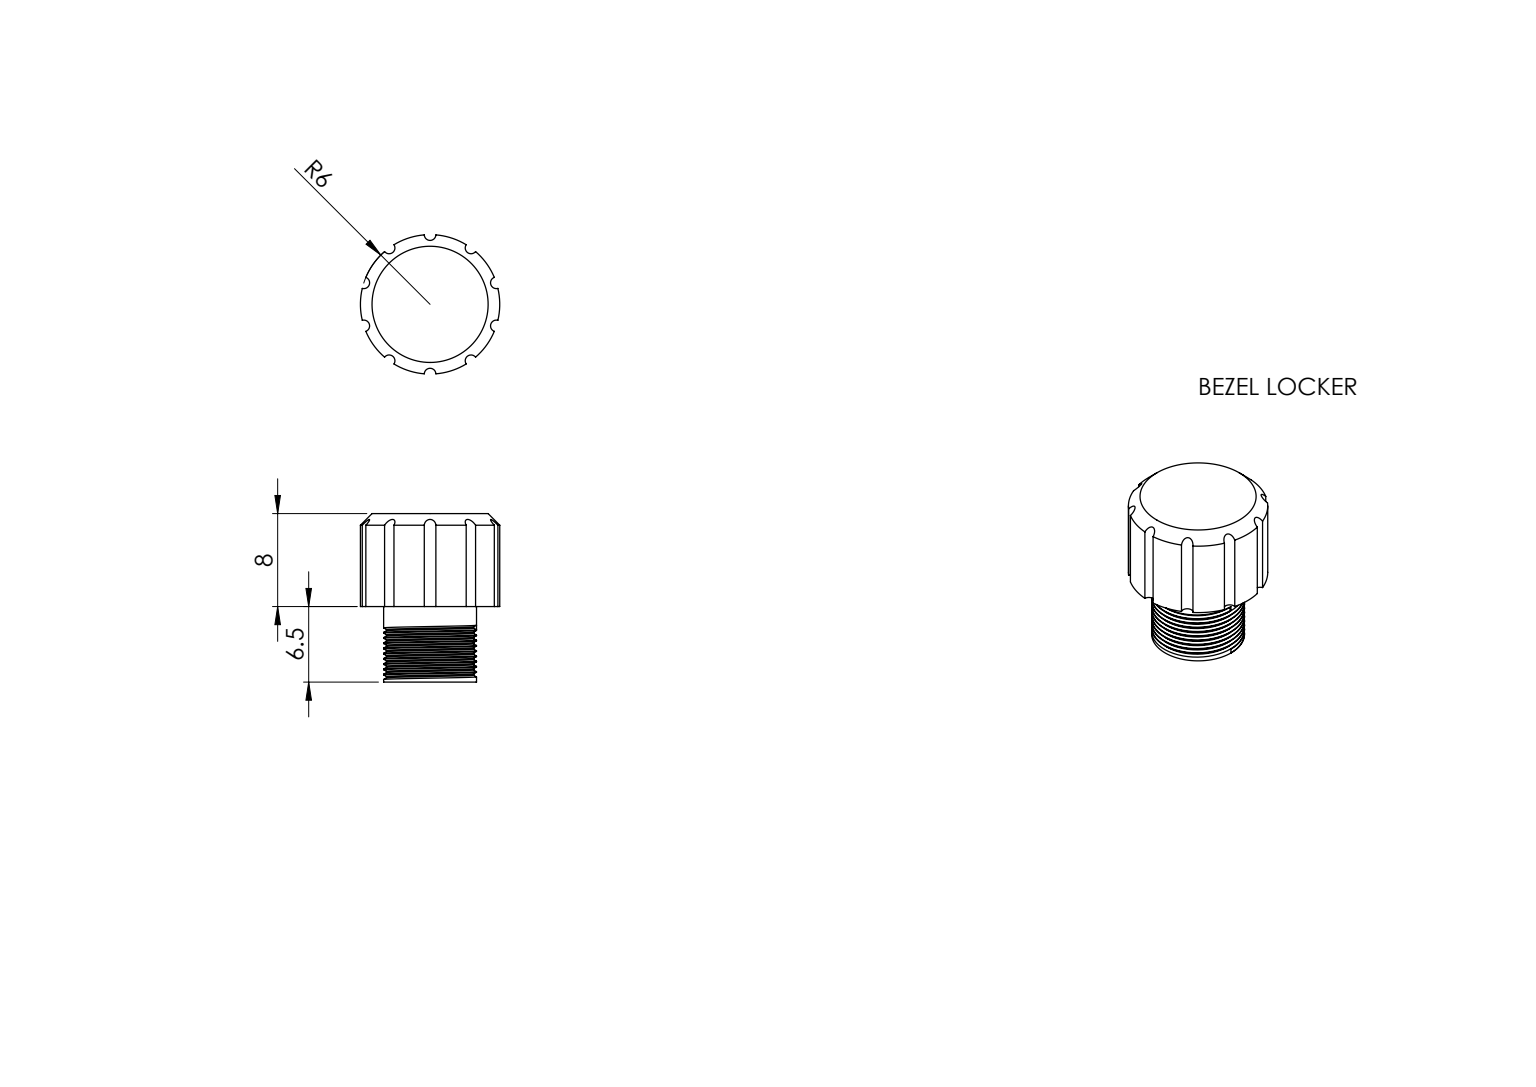
ISO-10303-21;
HEADER;
FILE_DESCRIPTION (('STEP AP214'),
    '1' );
FILE_NAME ('bezel locker.step',
    '2026-10-26T12:50:16',
    ( '' ),
    ( '' ),
    'SwSTEP 2.0',
    'SolidWorks 2026',
    '' );
FILE_SCHEMA (( 'AUTOMOTIVE_DESIGN' ));
ENDSEC;

DATA;
#10=DIRECTION ( 'NONE',  ( 0.000000000000000000, 0.000000000000000000, -1.000000000000000000 ) ) ;
#19=CARTESIAN_POINT ( 'NONE',  ( 3.469446951953614189E-15, 35.50000000000000711, 8.999999999999992895 ) ) ;
#32=VERTEX_POINT ( 'NONE', #17367 ) ;
#40=CARTESIAN_POINT ( 'NONE',  ( 7.901901826148023498E-15, 27.53124999877097068, 12.99999999999999112 ) ) ;
#46=CONICAL_SURFACE ( 'NONE', #10212, 5.000000000000000888, 0.7853981633974445042 ) ;
#53=CARTESIAN_POINT ( 'NONE',  ( -3.999999999999996447, 29.63124999877097210, 6.690598923241487306 ) ) ;
#61=ADVANCED_FACE ( 'NONE', ( #4267 ), #12239, .F. ) ;
#62=ORIENTED_EDGE ( 'NONE', *, *, #6026, .F. ) ;
#69=CARTESIAN_POINT ( 'NONE',  ( -3.756430356249997882, 29.45312499938549067, 11.16877607737301048 ) ) ;
#73=CARTESIAN_POINT ( 'NONE',  ( 4.000000000000002665, 27.21250000000000568, 11.30940107675849760 ) ) ;
#87=CARTESIAN_POINT ( 'NONE',  ( 3.756430356250004987, 25.19687499938549280, 8.999999999999992895 ) ) ;
#92=CARTESIAN_POINT ( 'NONE',  ( 4.006172263299091013E-15, 27.16562499938547859, 4.662447845253954171 ) ) ;
#93=ORIENTED_EDGE ( 'NONE', *, *, #14257, .T. ) ;
#101=CARTESIAN_POINT ( 'NONE',  ( 3.756430356250002323, 27.35312499938548569, 11.16877607737301226 ) ) ;
#113=EDGE_CURVE ( 'NONE', #22373, #14800, #20983, .T. ) ;
#114=DIRECTION ( 'NONE',  ( -0.000000000000000000, -1.000000000000000000, -0.000000000000000000 ) ) ;
#115=CARTESIAN_POINT ( 'NONE',  ( 3.718542035834364277E-15, 25.11250000000000782, 4.999999999999992006 ) ) ;
#118=CARTESIAN_POINT ( 'NONE',  ( -5.395002858709908367, 38.91217497027906802, 10.45656796931105426 ) ) ;
#121=AXIS2_PLACEMENT_3D ( 'NONE', #5758, #23946, #12025 ) ;
#123=CARTESIAN_POINT ( 'NONE',  ( 3.469446951953614189E-15, 35.50000000000000711, 4.999999999999992006 ) ) ;
#124=CARTESIAN_POINT ( 'NONE',  ( 3.370160183775990248, 38.97860908142764913, 13.37397733810513856 ) ) ;
#126=CARTESIAN_POINT ( 'NONE',  ( 2.000000000000005329, 26.81874999877097210, 5.535898384862238508 ) ) ;
#127=CARTESIAN_POINT ( 'NONE',  ( 3.469446951953614189E-15, 35.50000000000000711, 4.999999999999992006 ) ) ;
#139=CARTESIAN_POINT ( 'NONE',  ( -1.878215178124998275, 25.89062499938549067, 12.25316411605951927 ) ) ;
#144=EDGE_CURVE ( 'NONE', #7410, #22395, #341, .T. ) ;
#155=CARTESIAN_POINT ( 'NONE',  ( 1.071796769724497222, 28.00134618820329990, 12.99999999999998757 ) ) ;
#166=ORIENTED_EDGE ( 'NONE', *, *, #16755, .F. ) ;
#185=CARTESIAN_POINT ( 'NONE',  ( -1.878215178124994722, 25.40312499938548996, 5.746835883940462963 ) ) ;
#189=CARTESIAN_POINT ( 'NONE',  ( -3.999999999999996447, 29.23750000000001137, 6.690598923241487306 ) ) ;
#194=LINE ( 'NONE', #20580, #24770 ) ;
#196=FACE_OUTER_BOUND ( 'NONE', #24755, .T. ) ;
#200=CARTESIAN_POINT ( 'NONE',  ( -1.859271017917182139E-15, 26.46249999999999858, 4.999999999999991118 ) ) ;
#204=EDGE_CURVE ( 'NONE', #4422, #2251, #3256, .T. ) ;
#216=CARTESIAN_POINT ( 'NONE',  ( -1.878215178124999829, 26.90312499938548640, 12.25316411605951927 ) ) ;
#224=CARTESIAN_POINT ( 'NONE',  ( -3.756430356249998326, 28.10312499938548569, 11.16877607737301226 ) ) ;
#228=CARTESIAN_POINT ( 'NONE',  ( -3.999999999999999112, 28.35624999877097707, 11.30940107675849404 ) ) ;
#236=CARTESIAN_POINT ( 'NONE',  ( -3.999999999999996447, 26.51874999877097494, 8.999999999999992895 ) ) ;
#241=DIRECTION ( 'NONE',  ( -0.000000000000000000, -1.000000000000000000, -0.000000000000000000 ) ) ;
#247=CARTESIAN_POINT ( 'NONE',  ( -4.000000000000001776, 29.21874999877097068, 8.999999999999992895 ) ) ;
#251=CARTESIAN_POINT ( 'NONE',  ( 4.000000000000002665, 26.70624999877097849, 11.30940107675849760 ) ) ;
#264=CARTESIAN_POINT ( 'NONE',  ( 1.878215178125001605, 27.76562499938548711, 12.25316411605952283 ) ) ;
#302=DIRECTION ( 'NONE',  ( 0.000000000000000000, 0.000000000000000000, -1.000000000000000000 ) ) ;
#305=ORIENTED_EDGE ( 'NONE', *, *, #21565, .F. ) ;
#307=CARTESIAN_POINT ( 'NONE',  ( -3.756430356250002323, 27.31562499938548783, 11.16877607737301226 ) ) ;
#322=CARTESIAN_POINT ( 'NONE',  ( -3.999999999999996447, 28.86250000000000071, 11.30940107675849404 ) ) ;
#333=ORIENTED_EDGE ( 'NONE', *, *, #23959, .T. ) ;
#336=CARTESIAN_POINT ( 'NONE',  ( -1.878215178124998275, 28.25312499938548783, 12.25316411605951927 ) ) ;
#340=EDGE_CURVE ( 'NONE', #19215, #8133, #14856, .T. ) ;
#341=LINE ( 'NONE', #20331, #16761 ) ;
#345=VERTEX_POINT ( 'NONE', #10775 ) ;
#348=CARTESIAN_POINT ( 'NONE',  ( -1.878215178124999829, 29.04062499938549280, 12.25316411605951927 ) ) ;
#352=CIRCLE ( 'NONE', #6610, 6.000000000000000000 ) ;
#355=AXIS2_PLACEMENT_3D ( 'NONE', #19379, #17425, #11406 ) ;
#384=ADVANCED_FACE ( 'NONE', ( #5558 ), #46, .T. ) ;
#386=CARTESIAN_POINT ( 'NONE',  ( -1.878215178124998275, 25.55312499938549564, 12.25316411605951927 ) ) ;
#388=AXIS2_PLACEMENT_3D ( 'NONE', #11786, #19763, #1858 ) ;
#389=EDGE_CURVE ( 'NONE', #6543, #18698, #23590, .T. ) ;
#398=CARTESIAN_POINT ( 'NONE',  ( 3.918623196469464443, 31.50000000000000000, 4.456389954662531849 ) ) ;
#409=CARTESIAN_POINT ( 'NONE',  ( 2.000000000000003553, 27.71874999877097778, 5.535898384862238508 ) ) ;
#415=EDGE_LOOP ( 'NONE', ( #19879, #25527, #12734, #3697 ) ) ;
#418=FACE_OUTER_BOUND ( 'NONE', #25244, .T. ) ;
#445=CARTESIAN_POINT ( 'NONE',  ( -1.878215178124994722, 26.75312499938549138, 5.746835883940462963 ) ) ;
#458=CARTESIAN_POINT ( 'NONE',  ( 3.469446951953614189E-15, 39.50000000000000000, 8.999999999999992895 ) ) ;
#462=LINE ( 'NONE', #12609, #10063 ) ;
#463=DIRECTION ( 'NONE',  ( -0.000000000000000000, -1.000000000000000000, -0.000000000000000000 ) ) ;
#475=CARTESIAN_POINT ( 'NONE',  ( 5.255164635687713748, 38.99989214654019065, 10.62496012790605704 ) ) ;
#479=CARTESIAN_POINT ( 'NONE',  ( -1.878215178124998275, 28.10312499938548925, 5.746835883940462963 ) ) ;
#482=CARTESIAN_POINT ( 'NONE',  ( 3.469446951953614189E-15, 39.50000000000000000, 8.999999999999992895 ) ) ;
#486=VERTEX_POINT ( 'NONE', #5677 ) ;
#488=CARTESIAN_POINT ( 'NONE',  ( 1.878215178125003382, 28.36562499938548498, 5.746835883940462963 ) ) ;
#518=AXIS2_PLACEMENT_3D ( 'NONE', #19501, #15217, #9328 ) ;
#524=CARTESIAN_POINT ( 'NONE',  ( 1.487416814333745711E-14, 28.03750000000001208, 12.99999999999999289 ) ) ;
#525=CARTESIAN_POINT ( 'NONE',  ( 1.878215178125005158, 25.77812499938548996, 5.746835883940462963 ) ) ;
#530=CARTESIAN_POINT ( 'NONE',  ( -3.481870629348635671, 38.92501902593045315, 4.645898033751316270 ) ) ;
#556=AXIS2_PLACEMENT_3D ( 'NONE', #19, #15717, #3807 ) ;
#558=DIRECTION ( 'NONE',  ( 0.000000000000000000, 1.000000000000000000, 0.000000000000000000 ) ) ;
#578=CARTESIAN_POINT ( 'NONE',  ( -1.878215178124999829, 26.90312499938548640, 12.25316411605951927 ) ) ;
#587=STYLED_ITEM('',(#25907),#5394);
#600=CARTESIAN_POINT ( 'NONE',  ( -0.4995657836784015426, 38.49999999999999289, 3.020833333333323267 ) ) ;
#601=CARTESIAN_POINT ( 'NONE',  ( 4.000000000000002665, 25.80624999877096926, 11.30940107675849760 ) ) ;
#604=EDGE_CURVE ( 'NONE', #23841, #1729, #1999, .T. ) ;
#605=CARTESIAN_POINT ( 'NONE',  ( 5.563387625853419394, 38.77026726007181878, 10.37110993082982979 ) ) ;
#609=CARTESIAN_POINT ( 'NONE',  ( 3.756430356250002323, 27.46562499938548640, 11.16877607737301403 ) ) ;
#614=CARTESIAN_POINT ( 'NONE',  ( 3.526711513754818395, 29.50000000000000000, 4.145898033750289535 ) ) ;
#618=CARTESIAN_POINT ( 'NONE',  ( 3.756430356250004987, 27.84062499938548640, 8.999999999999992895 ) ) ;
#631=FACE_OUTER_BOUND ( 'NONE', #5269, .T. ) ;
#633=CARTESIAN_POINT ( 'NONE',  ( -3.999999999999998224, 25.61874999877097281, 8.999999999999992895 ) ) ;
#639=DIRECTION ( 'NONE',  ( 0.000000000000000000, 1.000000000000000000, -0.000000000000000000 ) ) ;
#656=DIRECTION ( 'NONE',  ( 0.000000000000000000, -1.000000000000000000, -0.000000000000000000 ) ) ;
#699=CARTESIAN_POINT ( 'NONE',  ( 3.756430356250004543, 28.81562499938548783, 11.16877607737301226 ) ) ;
#704=CARTESIAN_POINT ( 'NONE',  ( -1.071796769724485232, 27.77634618820331269, 4.999999999999992006 ) ) ;
#711=LINE ( 'NONE', #8815, #3315 ) ;
#718=CARTESIAN_POINT ( 'NONE',  ( 0.000000000000000000, 25.73124999877097352, 13.61880215351699874 ) ) ;
#719=CARTESIAN_POINT ( 'NONE',  ( 3.959305671612554781E-15, 35.50000000000000711, 12.99999999999999289 ) ) ;
#735=CARTESIAN_POINT ( 'NONE',  ( 3.756430356250003211, 26.04062499938548925, 8.999999999999992895 ) ) ;
#751=ORIENTED_EDGE ( 'NONE', *, *, #3136, .F. ) ;
#759=CARTESIAN_POINT ( 'NONE',  ( 4.000000000000001776, 29.89374999877097139, 8.999999999999992895 ) ) ;
#765=CARTESIAN_POINT ( 'NONE',  ( -3.756430356249996105, 25.44062499938548783, 6.831223922626973533 ) ) ;
#797=ORIENTED_EDGE ( 'NONE', *, *, #18776, .F. ) ;
#804=LINE ( 'NONE', #24741, #11411 ) ;
#810=DIRECTION ( 'NONE',  ( -0.000000000000000000, -1.000000000000000000, 0.000000000000000000 ) ) ;
#813=CARTESIAN_POINT ( 'NONE',  ( -3.999999999999996447, 29.63124999877097210, 6.690598923241487306 ) ) ;
#816=DIRECTION ( 'NONE',  ( 0.000000000000000000, 0.000000000000000000, 1.000000000000000000 ) ) ;
#819=CARTESIAN_POINT ( 'NONE',  ( 1.878215178125003382, 28.02812499938548996, 5.746835883940462963 ) ) ;
#847=CARTESIAN_POINT ( 'NONE',  ( -3.999999999999996447, 26.48124999877096997, 6.690598923241487306 ) ) ;
#849=CARTESIAN_POINT ( 'NONE',  ( 5.428131658003001903, 38.61087488181073724, 11.28411968614168615 ) ) ;
#855=VERTEX_POINT ( 'NONE', #17017 ) ;
#864=CARTESIAN_POINT ( 'NONE',  ( -3.756430356249996549, 26.67812499938548854, 6.831223922626973533 ) ) ;
#865=AXIS2_PLACEMENT_3D ( 'NONE', #18096, #5921, #4344 ) ;
#866=CARTESIAN_POINT ( 'NONE',  ( 1.071796769724492782, 26.44240381056766509, 4.999999999999989342 ) ) ;
#867=CARTESIAN_POINT ( 'NONE',  ( 3.756430356250002323, 28.25312499938548783, 11.16877607737301226 ) ) ;
#882=AXIS2_PLACEMENT_3D ( 'NONE', #14642, #16737, #24706 ) ;
#884=CARTESIAN_POINT ( 'NONE',  ( -3.999999999999996447, 25.65624999877097068, 11.30940107675849404 ) ) ;
#902=CARTESIAN_POINT ( 'NONE',  ( -3.756430356249994773, 28.17812499938548854, 8.999999999999992895 ) ) ;
#924=CARTESIAN_POINT ( 'NONE',  ( 4.648177544792955347E-16, 26.68750000000000711, 12.99999999999999289 ) ) ;
#930=VERTEX_POINT ( 'NONE', #7833 ) ;
#948=AXIS2_PLACEMENT_3D ( 'NONE', #2206, #241, #4289 ) ;
#958=AXIS2_PLACEMENT_3D ( 'NONE', #19324, #9263, #17252 ) ;
#960=ORIENTED_EDGE ( 'NONE', *, *, #11857, .T. ) ;
#981=ORIENTED_EDGE ( 'NONE', *, *, #3136, .T. ) ;
#982=CARTESIAN_POINT ( 'NONE',  ( 2.000000000000000000, 25.76874999877097139, 12.46410161513774817 ) ) ;
#996=LINE ( 'NONE', #14734, #15134 ) ;
#1000=CARTESIAN_POINT ( 'NONE',  ( -1.878215178124999829, 29.04062499938549280, 12.25316411605951927 ) ) ;
#1020=DIRECTION ( 'NONE',  ( -0.000000000000000000, -1.000000000000000000, -0.000000000000000000 ) ) ;
#1031=CARTESIAN_POINT ( 'NONE',  ( 3.756430356250004543, 28.81562499938548783, 11.16877607737301226 ) ) ;
#1035=EDGE_CURVE ( 'NONE', #18677, #23884, #21970, .T. ) ;
#1036=CARTESIAN_POINT ( 'NONE',  ( -3.100818392631252696, 38.96327129008100343, 4.412772063012910806 ) ) ;
#1054=EDGE_LOOP ( 'NONE', ( #15352, #6511, #21097, #21569 ) ) ;
#1063=( BOUNDED_SURFACE ( )  B_SPLINE_SURFACE ( 1, 2, ( 
 ( #4499, #12474, #18900, #2547, #4375, #12621, #12354, #10517, #18514, #718, #982, #601, #16550, #14846, #24780, #24255, #24509, #6591, #24638, #16670, #10766, #20594, #2680, #6726, #14718, #4778, #20723, #4895, #18755, #847, #8827, #6863, #12871, #11156, #21500, #11290, #17201, #15234, #13531, #5029, #25173, #22943, #11037, #23082, #11550, #16938, #23320, #23458, #9347, #23198, #21375, #9466, #19016, #13398, #15350, #3188, #5168, #19137, #24908, #21231, #19517, #13009, #7121, #9211, #7253, #1100, #25294, #7497, #13259, #3314, #15490, #20993, #6984, #15107, #3454, #5283, #17329, #11428, #14966, #9076, #3070, #17059, #5547, #19402, #7373, #3579, #25030, #8963, #19270, #1372, #13146, #5411, #21110, #1493, #1229, #17443, #25410, #13779, #8026, #21886, #9590, #21616, #23589, #11817, #25552, #10106, #13916, #13649, #15744, #23706, #4225, #5789, #25680, #53, #3699, #17712, #8155, #17576, #5670, #1887, #16135 ),
 ( #7883, #19655, #7637, #6179, #185, #11679, #24096, #9850, #15871, #14166, #25802, #22138, #9974, #1762, #9731, #17965, #21756, #16011, #3969, #15622, #7761, #3838, #19789, #17832, #18108, #11935, #23844, #5930, #19903, #12202, #2003, #23978, #6058, #14042, #22008, #1616, #4085, #12059, #20040, #2143, #445, #16259, #2658, #8414, #578, #12331, #10228, #24757, #24230, #6839, #20298, #18225, #18490, #8278, #6316, #307, #14550, #14823, #10346, #4476, #18729, #20698, #22795, #14312, #4872, #10620, #4610, #14692, #22274, #20172, #2392, #4354, #2273, #16403, #819, #22396, #16646, #18347, #22529, #12591, #12451, #24371, #20570, #2521, #8547, #6448, #14432, #10490, #20420, #16528, #24488, #6569, #18612, #8664, #8798, #699, #24613, #6698, #2779, #22672, #4759, #12728, #10742, #16787, #23397, #21179, #25488, #15806, #17276, #11366, #13477, #11495, #23265, #3641, #11753, #17511, #7574, #19732, #25241, #11227, #19345 ) ),
 .UNSPECIFIED., .F., .F., .F. ) 
 B_SPLINE_SURFACE_WITH_KNOTS ( ( 2, 2 ),
 ( 3, 2, 2, 2, 2, 2, 2, 2, 2, 2, 2, 2, 2, 2, 2, 2, 2, 2, 2, 2, 2, 2, 2, 2, 2, 2, 2, 2, 2, 2, 2, 2, 2, 2, 2, 2, 2, 2, 2, 2, 2, 2, 2, 2, 2, 2, 2, 2, 2, 2, 2, 2, 2, 2, 2, 2, 2, 2, 2, 2, 3 ),
 ( 0.000000000000000000, 1.000000000000000000 ),
 ( 0.000000000000000000, 0.01666666666666666644, 0.03333333333333333287, 0.05000000000000000278, 0.06666666666666666574, 0.08333333333333332871, 0.1000000000000000056, 0.1166666666666666685, 0.1333333333333333315, 0.1499999999999999944, 0.1666666666666666574, 0.1833333333333333204, 0.2000000000000000111, 0.2166666666666666741, 0.2333333333333333370, 0.2500000000000000000, 0.2666666666666666630, 0.2833333333333333259, 0.2999999999999999889, 0.3166666666666666519, 0.3333333333333333148, 0.3499999999999999778, 0.3666666666666666408, 0.3833333333333333592, 0.4000000000000000222, 0.4166666666666666852, 0.4333333333333333481, 0.4500000000000000111, 0.4666666666666666741, 0.4833333333333333370, 0.5000000000000000000, 0.5166666666666667185, 0.5333333333333333259, 0.5500000000000000444, 0.5666666666666666519, 0.5833333333333333703, 0.5999999999999999778, 0.6166666666666666963, 0.6333333333333333037, 0.6500000000000000222, 0.6666666666666666297, 0.6833333333333333481, 0.6999999999999999556, 0.7166666666666666741, 0.7333333333333332815, 0.7500000000000000000, 0.7666666666666667185, 0.7833333333333333259, 0.8000000000000000444, 0.8166666666666666519, 0.8333333333333333703, 0.8499999999999999778, 0.8666666666666666963, 0.8833333333333333037, 0.9000000000000000222, 0.9166666666666666297, 0.9333333333333333481, 0.9499999999999999556, 0.9666666666666666741, 0.9833333333333332815, 1.000000000000000000 ),
 .UNSPECIFIED. ) 
 GEOMETRIC_REPRESENTATION_ITEM ( )  RATIONAL_B_SPLINE_SURFACE ( (
 ( 1.000000000000000000, 0.8660254037844387076, 1.000000000000000000, 0.8660254037844387076, 1.000000000000000000, 0.8660254037844387076, 1.000000000000000000, 0.8660254037844387076, 1.000000000000000000, 0.8660254037844387076, 1.000000000000000000, 0.8660254037844387076, 1.000000000000000000, 0.8660254037844387076, 1.000000000000000000, 0.8660254037844387076, 1.000000000000000000, 0.8660254037844387076, 1.000000000000000000, 0.8660254037844387076, 1.000000000000000000, 0.8660254037844387076, 1.000000000000000000, 0.8660254037844387076, 1.000000000000000000, 0.8660254037844387076, 1.000000000000000000, 0.8660254037844387076, 1.000000000000000000, 0.8660254037844387076, 1.000000000000000000, 0.8660254037844387076, 1.000000000000000000, 0.8660254037844387076, 1.000000000000000000, 0.8660254037844387076, 1.000000000000000000, 0.8660254037844387076, 1.000000000000000000, 0.8660254037844387076, 1.000000000000000000, 0.8660254037844387076, 1.000000000000000000, 0.8660254037844387076, 1.000000000000000000, 0.8660254037844387076, 1.000000000000000000, 0.8660254037844387076, 1.000000000000000000, 0.8660254037844387076, 1.000000000000000000, 0.8660254037844387076, 1.000000000000000000, 0.8660254037844387076, 1.000000000000000000, 0.8660254037844387076, 1.000000000000000000, 0.8660254037844387076, 1.000000000000000000, 0.8660254037844387076, 1.000000000000000000, 0.8660254037844387076, 1.000000000000000000, 0.8660254037844387076, 1.000000000000000000, 0.8660254037844387076, 1.000000000000000000, 0.8660254037844387076, 1.000000000000000000, 0.8660254037844387076, 1.000000000000000000, 0.8660254037844387076, 1.000000000000000000, 0.8660254037844387076, 1.000000000000000000, 0.8660254037844387076, 1.000000000000000000, 0.8660254037844387076, 1.000000000000000000, 0.8660254037844387076, 1.000000000000000000, 0.8660254037844387076, 1.000000000000000000, 0.8660254037844387076, 1.000000000000000000, 0.8660254037844387076, 1.000000000000000000, 0.8660254037844387076, 1.000000000000000000, 0.8660254037844387076, 1.000000000000000000, 0.8660254037844387076, 1.000000000000000000, 0.8660254037844387076, 1.000000000000000000, 0.8660254037844387076, 1.000000000000000000, 0.8660254037844387076, 1.000000000000000000, 0.8660254037844387076, 1.000000000000000000, 0.8660254037844387076, 1.000000000000000000, 0.8660254037844387076, 1.000000000000000000, 0.8660254037844387076, 1.000000000000000000, 0.8660254037844387076, 1.000000000000000000, 0.8660254037844387076, 1.000000000000000000, 0.8660254037844387076, 1.000000000000000000, 0.8660254037844387076, 1.000000000000000000, 0.8660254037844387076, 1.000000000000000000, 0.8660254037844387076, 1.000000000000000000, 0.8660254037844387076, 1.000000000000000000),
 ( 1.000000000000000000, 0.8660254037844387076, 1.000000000000000000, 0.8660254037844387076, 1.000000000000000000, 0.8660254037844387076, 1.000000000000000000, 0.8660254037844387076, 1.000000000000000000, 0.8660254037844387076, 1.000000000000000000, 0.8660254037844387076, 1.000000000000000000, 0.8660254037844387076, 1.000000000000000000, 0.8660254037844387076, 1.000000000000000000, 0.8660254037844387076, 1.000000000000000000, 0.8660254037844387076, 1.000000000000000000, 0.8660254037844387076, 1.000000000000000000, 0.8660254037844387076, 1.000000000000000000, 0.8660254037844387076, 1.000000000000000000, 0.8660254037844387076, 1.000000000000000000, 0.8660254037844387076, 1.000000000000000000, 0.8660254037844387076, 1.000000000000000000, 0.8660254037844387076, 1.000000000000000000, 0.8660254037844387076, 1.000000000000000000, 0.8660254037844387076, 1.000000000000000000, 0.8660254037844387076, 1.000000000000000000, 0.8660254037844387076, 1.000000000000000000, 0.8660254037844387076, 1.000000000000000000, 0.8660254037844387076, 1.000000000000000000, 0.8660254037844387076, 1.000000000000000000, 0.8660254037844387076, 1.000000000000000000, 0.8660254037844387076, 1.000000000000000000, 0.8660254037844387076, 1.000000000000000000, 0.8660254037844387076, 1.000000000000000000, 0.8660254037844387076, 1.000000000000000000, 0.8660254037844387076, 1.000000000000000000, 0.8660254037844387076, 1.000000000000000000, 0.8660254037844387076, 1.000000000000000000, 0.8660254037844387076, 1.000000000000000000, 0.8660254037844387076, 1.000000000000000000, 0.8660254037844387076, 1.000000000000000000, 0.8660254037844387076, 1.000000000000000000, 0.8660254037844387076, 1.000000000000000000, 0.8660254037844387076, 1.000000000000000000, 0.8660254037844387076, 1.000000000000000000, 0.8660254037844387076, 1.000000000000000000, 0.8660254037844387076, 1.000000000000000000, 0.8660254037844387076, 1.000000000000000000, 0.8660254037844387076, 1.000000000000000000, 0.8660254037844387076, 1.000000000000000000, 0.8660254037844387076, 1.000000000000000000, 0.8660254037844387076, 1.000000000000000000, 0.8660254037844387076, 1.000000000000000000, 0.8660254037844387076, 1.000000000000000000, 0.8660254037844387076, 1.000000000000000000, 0.8660254037844387076, 1.000000000000000000, 0.8660254037844387076, 1.000000000000000000, 0.8660254037844387076, 1.000000000000000000, 0.8660254037844387076, 1.000000000000000000, 0.8660254037844387076, 1.000000000000000000, 0.8660254037844387076, 1.000000000000000000, 0.8660254037844387076, 1.000000000000000000, 0.8660254037844387076, 1.000000000000000000, 0.8660254037844387076, 1.000000000000000000, 0.8660254037844387076, 1.000000000000000000, 0.8660254037844387076, 1.000000000000000000) ) ) 
 REPRESENTATION_ITEM ( '' )  SURFACE ( )  );
#1073=DIRECTION ( 'NONE',  ( 0.000000000000000000, 0.000000000000000000, 1.000000000000000000 ) ) ;
#1082=ORIENTED_EDGE ( 'NONE', *, *, #23440, .T. ) ;
#1093=ADVANCED_FACE ( 'NONE', ( #14502 ), #10060, .T. ) ;
#1094=FACE_OUTER_BOUND ( 'NONE', #21501, .T. ) ;
#1100=CARTESIAN_POINT ( 'NONE',  ( -3.999999999999996447, 27.83124999877097139, 6.690598923241487306 ) ) ;
#1106=CARTESIAN_POINT ( 'NONE',  ( 1.878215178125001605, 28.77812499938549351, 12.25316411605952283 ) ) ;
#1114=CARTESIAN_POINT ( 'NONE',  ( -1.878215178124996498, 25.74062499938548854, 5.746835883940462963 ) ) ;
#1116=CARTESIAN_POINT ( 'NONE',  ( 3.756430356250003211, 28.29062499938548569, 8.999999999999992895 ) ) ;
#1129=DIRECTION ( 'NONE',  ( -0.000000000000000000, 1.000000000000000000, -0.000000000000000000 ) ) ;
#1139=VERTEX_POINT ( 'NONE', #19031 ) ;
#1147=CARTESIAN_POINT ( 'NONE',  ( 3.756430356250006319, 27.09062499938548285, 6.831223922626973533 ) ) ;
#1152=CARTESIAN_POINT ( 'NONE',  ( 4.648177544792955347E-16, 26.68750000000000711, 12.99999999999999289 ) ) ;
#1174=EDGE_CURVE ( 'NONE', #11752, #12276, #996, .T. ) ;
#1187=CARTESIAN_POINT ( 'NONE',  ( 0.000000000000000000, 29.78124999877097423, 12.99999999999999289 ) ) ;
#1191=CARTESIAN_POINT ( 'NONE',  ( 3.878215178125005380, 29.57031249969274356, 8.999999999999992895 ) ) ;
#1229=CARTESIAN_POINT ( 'NONE',  ( 2.000000000000000000, 28.91874999877097707, 12.46410161513774817 ) ) ;
#1240=AXIS2_PLACEMENT_3D ( 'NONE', #4577, #12555, #8637 ) ;
#1241=ORIENTED_EDGE ( 'NONE', *, *, #14257, .F. ) ;
#1244=CARTESIAN_POINT ( 'NONE',  ( -1.878215178124999829, 26.34062499938548996, 12.25316411605951927 ) ) ;
#1248=CARTESIAN_POINT ( 'NONE',  ( -1.999999999999998224, 25.75000000000000711, 12.46410161513774639 ) ) ;
#1279=DIRECTION ( 'NONE',  ( 0.000000000000000000, 1.000000000000000000, 0.000000000000000000 ) ) ;
#1280=CARTESIAN_POINT ( 'NONE',  ( -3.756430356249996105, 27.76562499938549422, 11.16877607737301226 ) ) ;
#1284=VECTOR ( 'NONE', #21794, 1000.000000000000000 ) ;
#1287=AXIS2_PLACEMENT_3D ( 'NONE', #614, #20207, #6093 ) ;
#1290=CARTESIAN_POINT ( 'NONE',  ( 2.000000000000003553, 29.12500000000000355, 5.535898384862238508 ) ) ;
#1320=FACE_OUTER_BOUND ( 'NONE', #10555, .T. ) ;
#1327=AXIS2_PLACEMENT_3D ( 'NONE', #16855, #1020, #18555 ) ;
#1331=DIRECTION ( 'NONE',  ( 0.000000000000000000, 1.000000000000000000, 0.000000000000000000 ) ) ;
#1341=CARTESIAN_POINT ( 'NONE',  ( 5.577813053751546416E-15, 25.33750000000000924, 12.99999999999999289 ) ) ;
#1350=ORIENTED_EDGE ( 'NONE', *, *, #3402, .F. ) ;
#1351=FACE_OUTER_BOUND ( 'NONE', #3967, .T. ) ;
#1358=VECTOR ( 'NONE', #8290, 1000.000000000000114 ) ;
#1363=CARTESIAN_POINT ( 'NONE',  ( 3.469446951953614189E-15, 35.50000000000000711, 8.999999999999992895 ) ) ;
#1372=CARTESIAN_POINT ( 'NONE',  ( -3.999999999999994671, 28.73124999877096997, 6.690598923241487306 ) ) ;
#1382=CARTESIAN_POINT ( 'NONE',  ( 3.469446951953614189E-15, 39.50000000000000000, 8.999999999999992895 ) ) ;
#1383=ORIENTED_EDGE ( 'NONE', *, *, #9460, .T. ) ;
#1386=CARTESIAN_POINT ( 'NONE',  ( 0.000000000000000000, 27.72812499938548569, 13.33755215474603162 ) ) ;
#1389=CARTESIAN_POINT ( 'NONE',  ( 1.878215178125003382, 28.36562499938548498, 5.746835883940462963 ) ) ;
#1398=CARTESIAN_POINT ( 'NONE',  ( -3.999999999999994671, 26.93124999877097281, 6.690598923241487306 ) ) ;
#1410=CARTESIAN_POINT ( 'NONE',  ( 3.756430356250004099, 25.74062499938548854, 6.831223922626973533 ) ) ;
#1411=ORIENTED_EDGE ( 'NONE', *, *, #13393, .F. ) ;
#1419=CARTESIAN_POINT ( 'NONE',  ( -1.878215178124998275, 27.35312499938548925, 12.25316411605951927 ) ) ;
#1431=ORIENTED_EDGE ( 'NONE', *, *, #11857, .F. ) ;
#1435=ADVANCED_FACE ( 'NONE', ( #14416 ), #20400, .T. ) ;
#1439=ORIENTED_EDGE ( 'NONE', *, *, #5014, .F. ) ;
#1443=EDGE_LOOP ( 'NONE', ( #4353, #16270, #22985, #14828, #6396, #3255 ) ) ;
#1486=ADVANCED_FACE ( 'NONE', ( #14531 ), #16900, .T. ) ;
#1493=CARTESIAN_POINT ( 'NONE',  ( 2.003086131649545506E-15, 28.88124999877097210, 13.61880215351699874 ) ) ;
#1496=DIRECTION ( 'NONE',  ( 0.000000000000000000, 0.000000000000000000, 1.000000000000000000 ) ) ;
#1500=EDGE_CURVE ( 'NONE', #6543, #19882, #20943, .T. ) ;
#1503=VERTEX_POINT ( 'NONE', #6819 ) ;
#1507=CARTESIAN_POINT ( 'NONE',  ( 3.756430356250002323, 27.80312499938548854, 11.16877607737301403 ) ) ;
#1511=CARTESIAN_POINT ( 'NONE',  ( 6.009258394948636914E-15, 26.01250000000000284, 4.381197846482986158 ) ) ;
#1514=CARTESIAN_POINT ( 'NONE',  ( -3.918623196469422698, 38.49999999999999289, 13.54361004533748059 ) ) ;
#1533=VERTEX_POINT ( 'NONE', #18708 ) ;
#1538=CARTESIAN_POINT ( 'NONE',  ( 1.878215178125003382, 29.67812499938549209, 12.25316411605952283 ) ) ;
#1545=CARTESIAN_POINT ( 'NONE',  ( 4.000000000000005329, 26.83750000000000213, 6.690598923241489970 ) ) ;
#1549=PLANE ( 'NONE',  #5781 ) ;
#1557=CARTESIAN_POINT ( 'NONE',  ( 3.918623196469491976, 38.49999999999999289, 13.54361004533742907 ) ) ;
#1571=CARTESIAN_POINT ( 'NONE',  ( -3.999999999999996447, 27.92500000000000426, 8.999999999999992895 ) ) ;
#1593=( BOUNDED_CURVE ( )  B_SPLINE_CURVE ( 2, ( #15644, #17088, #5190, #1398, #23610, #7280, #23108, #9485, #15257 ),
 .UNSPECIFIED., .F., .F. ) 
 B_SPLINE_CURVE_WITH_KNOTS ( ( 3, 2, 2, 2, 3 ),
 ( 0.3250000000000000111, 0.3333333333333333148, 0.3499999999999999778, 0.3666666666666666408, 0.3750000000000000000 ),
 .UNSPECIFIED. ) 
 CURVE ( )  GEOMETRIC_REPRESENTATION_ITEM ( )  RATIONAL_B_SPLINE_CURVE ( ( 0.9330127018922194093, 0.9330127018922196314, 1.000000000000000000, 0.8660254037844387076, 1.000000000000000000, 0.8660254037844387076, 1.000000000000000000, 0.9330127018922194093, 0.9330127018922194093 ) ) 
 REPRESENTATION_ITEM ( '' )  );
#1605=ADVANCED_FACE ( 'NONE', ( #8220 ), #13982, .F. ) ;
#1611=EDGE_CURVE ( 'NONE', #2153, #19796, #22459, .T. ) ;
#1613=CARTESIAN_POINT ( 'NONE',  ( 2.000000000000005329, 28.22500000000000497, 5.535898384862238508 ) ) ;
#1616=CARTESIAN_POINT ( 'NONE',  ( 3.756430356250000546, 26.56562499938548783, 11.16877607737301226 ) ) ;
#1625=CARTESIAN_POINT ( 'NONE',  ( 1.071796769724495224, 25.09240381056766722, 4.999999999999992895 ) ) ;
#1629=CARTESIAN_POINT ( 'NONE',  ( 3.481718437949647083, 38.92511481668519480, 4.645898033752395406 ) ) ;
#1631=CARTESIAN_POINT ( 'NONE',  ( 3.756430356250003211, 28.74062499938548498, 8.999999999999992895 ) ) ;
#1633=CARTESIAN_POINT ( 'NONE',  ( 4.000000000000005329, 26.38750000000000639, 6.690598923241489970 ) ) ;
#1652=CARTESIAN_POINT ( 'NONE',  ( 2.000000000000000000, 25.76874999877097139, 12.46410161513774817 ) ) ;
#1668=CARTESIAN_POINT ( 'NONE',  ( 3.756430356250004987, 25.14062499938548356, 8.999999999999992895 ) ) ;
#1676=CARTESIAN_POINT ( 'NONE',  ( 4.000000000000005329, 29.05000000000000426, 8.999999999999992895 ) ) ;
#1695=CARTESIAN_POINT ( 'NONE',  ( 6.972266317189432034E-15, 28.65624999877097423, 4.999999999999992006 ) ) ;
#1727=CARTESIAN_POINT ( 'NONE',  ( 3.469446951953614189E-15, 35.50000000000000711, 8.999999999999992895 ) ) ;
#1729=VERTEX_POINT ( 'NONE', #20262 ) ;
#1746=VECTOR ( 'NONE', #2061, 1000.000000000000000 ) ;
#1753=CARTESIAN_POINT ( 'NONE',  ( 1.071796769724488563, 29.08615380933863648, 4.999999999999988454 ) ) ;
#1761=ORIENTED_EDGE ( 'NONE', *, *, #2756, .F. ) ;
#1762=CARTESIAN_POINT ( 'NONE',  ( 3.756430356250004543, 25.74062499938548498, 6.831223922626973533 ) ) ;
#1776=CARTESIAN_POINT ( 'NONE',  ( 1.878215178125006934, 27.91562499938549280, 5.746835883940462963 ) ) ;
#1778=CARTESIAN_POINT ( 'NONE',  ( 2.000000000000000000, 27.62500000000000355, 12.46410161513774817 ) ) ;
#1789=EDGE_CURVE ( 'NONE', #2251, #13124, #15580, .T. ) ;
#1806=CARTESIAN_POINT ( 'NONE',  ( 1.878215178125003382, 25.66562499938548214, 5.746835883940462963 ) ) ;
#1816=DIRECTION ( 'NONE',  ( 0.000000000000000000, 1.000000000000000000, -0.000000000000000000 ) ) ;
#1826=CARTESIAN_POINT ( 'NONE',  ( -1.071796769724485676, 26.21740381056767077, 12.99999999999999467 ) ) ;
#1828=ORIENTED_EDGE ( 'NONE', *, *, #6632, .F. ) ;
#1843=CARTESIAN_POINT ( 'NONE',  ( 1.878215178125003382, 27.01562499938548711, 5.746835883940462963 ) ) ;
#1858=DIRECTION ( 'NONE',  ( 0.000000000000000000, 0.000000000000000000, 1.000000000000000000 ) ) ;
#1879=CARTESIAN_POINT ( 'NONE',  ( 5.112995299272250684E-15, 25.56250000000000711, 4.999999999999992006 ) ) ;
#1882=DIRECTION ( 'NONE',  ( -0.000000000000000000, -1.000000000000000000, -0.000000000000000000 ) ) ;
#1886=EDGE_LOOP ( 'NONE', ( #10348, #2305, #20236, #25362 ) ) ;
#1887=CARTESIAN_POINT ( 'NONE',  ( 4.000000000000000888, 29.85624999877096997, 11.30940107675849760 ) ) ;
#1895=CARTESIAN_POINT ( 'NONE',  ( 9.296355089585910693E-16, 26.18124999877096926, 12.99999999999999289 ) ) ;
#1899=( BOUNDED_CURVE ( )  B_SPLINE_CURVE ( 2, ( #11750, #22065, #19966, #5728, #7956, #19729, #4154, #1826, #8094 ),
 .UNSPECIFIED., .F., .F. ) 
 B_SPLINE_CURVE_WITH_KNOTS ( ( 3, 2, 2, 2, 3 ),
 ( 0.2250000000000000056, 0.2333333333333333370, 0.2500000000000000000, 0.2666666666666666630, 0.2750000000000000222 ),
 .UNSPECIFIED. ) 
 CURVE ( )  GEOMETRIC_REPRESENTATION_ITEM ( )  RATIONAL_B_SPLINE_CURVE ( ( 0.9330127018922194093, 0.9330127018922194093, 1.000000000000000000, 0.8660254037844387076, 1.000000000000000000, 0.8660254037844387076, 1.000000000000000000, 0.9330127018922191873, 0.9330127018922194093 ) ) 
 REPRESENTATION_ITEM ( '' )  );
#1901=CARTESIAN_POINT ( 'NONE',  ( 3.756430356250004987, 27.84062499938548640, 8.999999999999992895 ) ) ;
#1902=CARTESIAN_POINT ( 'NONE',  ( 2.006336132164985451E-12, 39.00000000001113420, 3.500000000010202061 ) ) ;
#1903=CARTESIAN_POINT ( 'NONE',  ( 2.000000000000003553, 27.32500000000000995, 5.535898384862238508 ) ) ;
#1916=CARTESIAN_POINT ( 'NONE',  ( 4.648177544792954952E-15, 25.73124999877097707, 12.99999999999999289 ) ) ;
#1928=CARTESIAN_POINT ( 'NONE',  ( 3.756430356250002323, 26.45312499938549067, 11.16877607737301226 ) ) ;
#1941=CARTESIAN_POINT ( 'NONE',  ( -5.618699665603582361, 38.72260848564139479, 10.34687723573376594 ) ) ;
#1942=CARTESIAN_POINT ( 'NONE',  ( 5.501714610360307844, 38.82806989278485332, 7.617651621319569522 ) ) ;
#1950=CARTESIAN_POINT ( 'NONE',  ( 1.071796769724497222, 28.63615380933864429, 4.999999999999992895 ) ) ;
#1959=CARTESIAN_POINT ( 'NONE',  ( 8.012344526598182026E-15, 27.05312499938548854, 4.662447845253954171 ) ) ;
#1969=CARTESIAN_POINT ( 'NONE',  ( 1.071796769724496334, 27.79240381056767362, 4.999999999999992895 ) ) ;
#1983=ORIENTED_EDGE ( 'NONE', *, *, #340, .F. ) ;
#1999=( BOUNDED_CURVE ( )  B_SPLINE_CURVE ( 2, ( #3978, #22404, #8038, #17843, #21895, #20180, #13927, #19797, #1895 ),
 .UNSPECIFIED., .F., .F. ) 
 B_SPLINE_CURVE_WITH_KNOTS ( ( 3, 2, 2, 2, 3 ),
 ( 0.1250000000000000000, 0.1333333333333333315, 0.1499999999999999944, 0.1666666666666666574, 0.1749999999999999889 ),
 .UNSPECIFIED. ) 
 CURVE ( )  GEOMETRIC_REPRESENTATION_ITEM ( )  RATIONAL_B_SPLINE_CURVE ( ( 0.9330127018922194093, 0.9330127018922194093, 1.000000000000000000, 0.8660254037844387076, 1.000000000000000000, 0.8660254037844387076, 1.000000000000000000, 0.9330127018922194093, 0.9330127018922194093 ) ) 
 REPRESENTATION_ITEM ( '' )  );
#2003=CARTESIAN_POINT ( 'NONE',  ( -3.756430356249994773, 26.37812499938548783, 8.999999999999992895 ) ) ;
#2009=CARTESIAN_POINT ( 'NONE',  ( 3.469446951953614189E-15, 31.50000000000000000, 8.999999999999992895 ) ) ;
#2015=ORIENTED_EDGE ( 'NONE', *, *, #20840, .T. ) ;
#2016=CARTESIAN_POINT ( 'NONE',  ( 0.4451413195716044102, 38.71736240459208034, 14.76550166049843149 ) ) ;
#2022=CARTESIAN_POINT ( 'NONE',  ( 4.000000000000000888, 26.31250000000000711, 11.30940107675849760 ) ) ;
#2030=CARTESIAN_POINT ( 'NONE',  ( 3.756430356250004987, 29.64062499938548711, 8.999999999999992895 ) ) ;
#2041=CARTESIAN_POINT ( 'NONE',  ( -3.756430356249996549, 27.27812499938548996, 8.999999999999992895 ) ) ;
#2047=EDGE_LOOP ( 'NONE', ( #7063, #21624, #23983, #13118 ) ) ;
#2050=CARTESIAN_POINT ( 'NONE',  ( 1.878215178125005158, 28.81562499938548783, 5.746835883940462963 ) ) ;
#2060=DIRECTION ( 'NONE',  ( 0.000000000000000000, 0.000000000000000000, 1.000000000000000000 ) ) ;
#2061=DIRECTION ( 'NONE',  ( -0.000000000000000000, -1.000000000000000000, -0.000000000000000000 ) ) ;
#2063=CARTESIAN_POINT ( 'NONE',  ( -3.110308778861273105, 38.49999999999999289, 14.13088484572967118 ) ) ;
#2066=CARTESIAN_POINT ( 'NONE',  ( -5.201336420084783363, 38.97860908142765624, 10.85357947325328176 ) ) ;
#2069=AXIS2_PLACEMENT_3D ( 'NONE', #25572, #23104, #3093 ) ;
#2082=EDGE_CURVE ( 'NONE', #15046, #10411, #11305, .T. ) ;
#2088=CARTESIAN_POINT ( 'NONE',  ( -3.756430356249996549, 27.61562499938548143, 8.999999999999992895 ) ) ;
#2109=ORIENTED_EDGE ( 'NONE', *, *, #21512, .F. ) ;
#2126=DIRECTION ( 'NONE',  ( -0.000000000000000000, -1.000000000000000000, -0.000000000000000000 ) ) ;
#2128=EDGE_CURVE ( 'NONE', #23884, #11133, #10823, .T. ) ;
#2138=CYLINDRICAL_SURFACE ( 'NONE', #3780, 4.000000000000000000 ) ;
#2143=CARTESIAN_POINT ( 'NONE',  ( 4.006172263299091013E-15, 26.71562499938548996, 4.662447845253954171 ) ) ;
#2153=VERTEX_POINT ( 'NONE', #16671 ) ;
#2159=CARTESIAN_POINT ( 'NONE',  ( 2.000000000000000000, 28.52500000000000924, 12.46410161513774817 ) ) ;
#2162=VECTOR ( 'NONE', #14829, 1000.000000000000000 ) ;
#2175=VERTEX_POINT ( 'NONE', #24639 ) ;
#2178=CARTESIAN_POINT ( 'NONE',  ( -3.756430356249996549, 26.34062499938548285, 6.831223922626973533 ) ) ;
#2185=DIRECTION ( 'NONE',  ( 0.000000000000000000, 0.000000000000000000, 1.000000000000000000 ) ) ;
#2187=CARTESIAN_POINT ( 'NONE',  ( 3.756430356250002323, 27.80312499938548854, 11.16877607737301226 ) ) ;
#2189=AXIS2_PLACEMENT_3D ( 'NONE', #23804, #15712, #12018 ) ;
#2195=CARTESIAN_POINT ( 'NONE',  ( -1.999999999999994893, 28.24374999877096926, 5.535898384862237620 ) ) ;
#2206=CARTESIAN_POINT ( 'NONE',  ( 3.469446951953614189E-15, 39.50000000000000000, 8.999999999999992895 ) ) ;
#2207=CARTESIAN_POINT ( 'NONE',  ( 5.442264176411883980, 38.59882996731582239, 6.718392883288001549 ) ) ;
#2221=EDGE_LOOP ( 'NONE', ( #25871, #19213, #10345, #5237 ) ) ;
#2226=CARTESIAN_POINT ( 'NONE',  ( -1.878215178124996498, 26.19062499938548783, 5.746835883940462963 ) ) ;
#2236=CARTESIAN_POINT ( 'NONE',  ( 2.000000000000000000, 26.21874999877097423, 12.46410161513774817 ) ) ;
#2241=EDGE_CURVE ( 'NONE', #5871, #345, #15594, .T. ) ;
#2248=ORIENTED_EDGE ( 'NONE', *, *, #24328, .T. ) ;
#2249=ORIENTED_EDGE ( 'NONE', *, *, #1789, .F. ) ;
#2251=VERTEX_POINT ( 'NONE', #21208 ) ;
#2259=FACE_OUTER_BOUND ( 'NONE', #17250, .T. ) ;
#2273=CARTESIAN_POINT ( 'NONE',  ( 3.756430356250004987, 27.95312499938548711, 8.999999999999992895 ) ) ;
#2282=CARTESIAN_POINT ( 'NONE',  ( -0.3338636427494882097, 38.86740601410824780, 14.62281502694621871 ) ) ;
#2290=CARTESIAN_POINT ( 'NONE',  ( 3.469446951953614189E-15, 35.50000000000000711, 8.999999999999992895 ) ) ;
#2299=ORIENTED_EDGE ( 'NONE', *, *, #18717, .T. ) ;
#2303=CARTESIAN_POINT ( 'NONE',  ( 3.756430356250006319, 27.99062499938548854, 6.831223922626973533 ) ) ;
#2305=ORIENTED_EDGE ( 'NONE', *, *, #340, .T. ) ;
#2313=CARTESIAN_POINT ( 'NONE',  ( -3.756430356249998326, 27.20312499938549067, 11.16877607737301226 ) ) ;
#2346=CARTESIAN_POINT ( 'NONE',  ( 3.756430356250004543, 26.19062499938549138, 6.831223922626973533 ) ) ;
#2375=ORIENTED_EDGE ( 'NONE', *, *, #16611, .F. ) ;
#2378=EDGE_CURVE ( 'NONE', #930, #4422, #11895, .T. ) ;
#2389=CARTESIAN_POINT ( 'NONE',  ( 4.000000000000003553, 25.39374999877097494, 8.999999999999992895 ) ) ;
#2392=CARTESIAN_POINT ( 'NONE',  ( 1.878215178125001605, 27.87812499938548783, 12.25316411605952283 ) ) ;
#2402=CARTESIAN_POINT ( 'NONE',  ( 1.878215178125006934, 29.26562499938549067, 5.746835883940462963 ) ) ;
#2405=CARTESIAN_POINT ( 'NONE',  ( -3.999999999999996447, 28.37500000000000355, 8.999999999999992895 ) ) ;
#2408=CARTESIAN_POINT ( 'NONE',  ( -0.3342655765624286679, 38.86701176172695682, 3.376814578616960993 ) ) ;
#2417=CARTESIAN_POINT ( 'NONE',  ( 3.756430356250003211, 28.40312499938548640, 8.999999999999992895 ) ) ;
#2421=( BOUNDED_CURVE ( )  B_SPLINE_CURVE ( 2, ( #18067, #19869, #2236, #15975, #15710, #17798, #25764, #6276, #7845 ),
 .UNSPECIFIED., .F., .F. ) 
 B_SPLINE_CURVE_WITH_KNOTS ( ( 3, 2, 2, 2, 3 ),
 ( 0.1749999999999999889, 0.1833333333333333204, 0.2000000000000000111, 0.2166666666666666741, 0.2250000000000000056 ),
 .UNSPECIFIED. ) 
 CURVE ( )  GEOMETRIC_REPRESENTATION_ITEM ( )  RATIONAL_B_SPLINE_CURVE ( ( 0.9330127018922194093, 0.9330127018922194093, 1.000000000000000000, 0.8660254037844387076, 1.000000000000000000, 0.8660254037844387076, 1.000000000000000000, 0.9330127018922194093, 0.9330127018922194093 ) ) 
 REPRESENTATION_ITEM ( '' )  );
#2422=CARTESIAN_POINT ( 'NONE',  ( 3.526711513754840599, 38.89679573513954125, 4.645898033750303746 ) ) ;
#2425=ORIENTED_EDGE ( 'NONE', *, *, #14687, .F. ) ;
#2428=CARTESIAN_POINT ( 'NONE',  ( 3.756430356250003211, 27.39062499938548711, 8.999999999999992895 ) ) ;
#2449=ORIENTED_EDGE ( 'NONE', *, *, #113, .F. ) ;
#2450=CARTESIAN_POINT ( 'NONE',  ( 3.253724281355068545E-15, 25.50624999877097210, 4.999999999999992006 ) ) ;
#2454=CARTESIAN_POINT ( 'NONE',  ( 3.469446951953614189E-15, 25.00000000000000000, 8.999999999999992895 ) ) ;
#2469=EDGE_CURVE ( 'NONE', #486, #6625, #14572, .T. ) ;
#2480=EDGE_CURVE ( 'NONE', #15689, #16757, #16751, .T. ) ;
#2481=B_SPLINE_CURVE_WITH_KNOTS ( 'NONE', 3,
 ( #5805, #23858, #25565, #19915, #7896, #11692, #9741, #13543, #7773, #17454, #17720, #19528, #1629, #21897 ),
 .UNSPECIFIED., .F., .F.,
 ( 4, 2, 2, 2, 2, 2, 4 ),
 ( 2.789812634828778690E-07, 0.0003151273862689746037, 0.0006299757912744662633, 0.0007873999937772171347, 0.0009448241962799682229, 0.001102248398782719203, 0.001259672601285470291 ),
 .UNSPECIFIED. ) ;
#2482=CARTESIAN_POINT ( 'NONE',  ( -1.071796769724482123, 27.56740381056766864, 12.99999999999999645 ) ) ;
#2487=ORIENTED_EDGE ( 'NONE', *, *, #2756, .T. ) ;
#2488=CARTESIAN_POINT ( 'NONE',  ( -5.840899737312981621, 34.50000000000000000, 7.627451181685283466 ) ) ;
#2519=ORIENTED_EDGE ( 'NONE', *, *, #23305, .T. ) ;
#2521=CARTESIAN_POINT ( 'NONE',  ( 3.756430356250000546, 28.36562499938549564, 11.16877607737301226 ) ) ;
#2525=CARTESIAN_POINT ( 'NONE',  ( -3.918623196469422698, 34.50000000000000000, 13.54361004533748059 ) ) ;
#2527=CARTESIAN_POINT ( 'NONE',  ( -1.999999999999998224, 28.30000000000000426, 5.535898384862237620 ) ) ;
#2539=CARTESIAN_POINT ( 'NONE',  ( 2.000000000000003553, 29.12500000000000355, 5.535898384862238508 ) ) ;
#2541=VECTOR ( 'NONE', #10189, 1000.000000000000000 ) ;
#2547=CARTESIAN_POINT ( 'NONE',  ( 4.006172263299091013E-15, 25.50624999877097920, 4.381197846482986158 ) ) ;
#2552=CARTESIAN_POINT ( 'NONE',  ( 5.621027209102163802, 38.71721868403345468, 10.35826165063589777 ) ) ;
#2556=CARTESIAN_POINT ( 'NONE',  ( -3.756430356249997882, 27.72812499938548569, 8.999999999999992895 ) ) ;
#2561=DIRECTION ( 'NONE',  ( -0.000000000000000000, 1.000000000000000000, -0.000000000000000000 ) ) ;
#2566=CARTESIAN_POINT ( 'NONE',  ( 3.756430356250003211, 26.94062499938548783, 8.999999999999992895 ) ) ;
#2574=( BOUNDED_CURVE ( )  B_SPLINE_CURVE ( 2, ( #15669, #5847, #2195, #15785, #8200, #228, #23636, #25725, #5714 ),
 .UNSPECIFIED., .F., .F. ) 
 B_SPLINE_CURVE_WITH_KNOTS ( ( 3, 2, 2, 2, 3 ),
 ( 0.6250000000000000000, 0.6333333333333333037, 0.6500000000000000222, 0.6666666666666666297, 0.6750000000000000444 ),
 .UNSPECIFIED. ) 
 CURVE ( )  GEOMETRIC_REPRESENTATION_ITEM ( )  RATIONAL_B_SPLINE_CURVE ( ( 0.9330127018922194093, 0.9330127018922194093, 1.000000000000000000, 0.8660254037844387076, 1.000000000000000000, 0.8660254037844387076, 1.000000000000000000, 0.9330127018922189652, 0.9330127018922194093 ) ) 
 REPRESENTATION_ITEM ( '' )  );
#2597=DIRECTION ( 'NONE',  ( 0.000000000000000000, 0.000000000000000000, 1.000000000000000000 ) ) ;
#2606=ADVANCED_FACE ( 'NONE', ( #2874 ), #8518, .T. ) ;
#2622=CARTESIAN_POINT ( 'NONE',  ( -1.071796769724485232, 27.38259618943233775, 4.999999999999992006 ) ) ;
#2634=EDGE_CURVE ( 'NONE', #15214, #10104, #12507, .T. ) ;
#2639=AXIS2_PLACEMENT_3D ( 'NONE', #5729, #9666, #17649 ) ;
#2647=AXIS2_PLACEMENT_3D ( 'NONE', #15781, #24015, #19563 ) ;
#2652=CARTESIAN_POINT ( 'NONE',  ( -1.071796769724488785, 28.86115380933863861, 12.99999999999999289 ) ) ;
#2658=CARTESIAN_POINT ( 'NONE',  ( -3.756430356249996549, 26.82812499938549067, 8.999999999999992895 ) ) ;
#2662=EDGE_LOOP ( 'NONE', ( #13155, #20391, #24862, #18260 ) ) ;
#2664=EDGE_LOOP ( 'NONE', ( #12172, #8183, #18204, #6376 ) ) ;
#2679=DIRECTION ( 'NONE',  ( 0.000000000000000000, 0.000000000000000000, 1.000000000000000000 ) ) ;
#2680=CARTESIAN_POINT ( 'NONE',  ( 2.000000000000000000, 26.21874999877097423, 12.46410161513774817 ) ) ;
#2683=CARTESIAN_POINT ( 'NONE',  ( 5.451523067058389849, 38.86679461760645182, 10.41960775444208842 ) ) ;
#2691=CYLINDRICAL_SURFACE ( 'NONE', #4972, 6.000000000000000888 ) ;
#2699=CARTESIAN_POINT ( 'NONE',  ( -3.756430356249998326, 25.85312499938549635, 11.16877607737301226 ) ) ;
#2734=( BOUNDED_CURVE ( )  B_SPLINE_CURVE ( 2, ( #19894, #21493, #13764, #3828, #19645, #15614, #23968, #16000, #40 ),
 .UNSPECIFIED., .F., .F. ) 
 B_SPLINE_CURVE_WITH_KNOTS ( ( 3, 2, 2, 2, 3 ),
 ( 0.4250000000000000444, 0.4333333333333333481, 0.4500000000000000111, 0.4666666666666666741, 0.4750000000000000333 ),
 .UNSPECIFIED. ) 
 CURVE ( )  GEOMETRIC_REPRESENTATION_ITEM ( )  RATIONAL_B_SPLINE_CURVE ( ( 0.9330127018922194093, 0.9330127018922196314, 1.000000000000000000, 0.8660254037844387076, 1.000000000000000000, 0.8660254037844387076, 1.000000000000000000, 0.9330127018922191873, 0.9330127018922194093 ) ) 
 REPRESENTATION_ITEM ( '' )  );
#2750=CARTESIAN_POINT ( 'NONE',  ( 5.112995299272250684E-15, 27.75624999877097565, 4.999999999999992006 ) ) ;
#2753=VERTEX_POINT ( 'NONE', #21444 ) ;
#2756=EDGE_CURVE ( 'NONE', #14800, #4850, #4597, .T. ) ;
#2773=CARTESIAN_POINT ( 'NONE',  ( -1.071796769724483456, 28.67634618820330772, 4.999999999999992006 ) ) ;
#2776=DIRECTION ( 'NONE',  ( 0.000000000000000000, 1.000000000000000000, -0.000000000000000000 ) ) ;
#2779=CARTESIAN_POINT ( 'NONE',  ( 1.878215178125008489, 28.92812499938549209, 5.746835883940462963 ) ) ;
#2801=EDGE_CURVE ( 'NONE', #22370, #19772, #25694, .T. ) ;
#2805=CARTESIAN_POINT ( 'NONE',  ( 5.297476235640267817, 38.97860908142764913, 10.55769154565112622 ) ) ;
#2808=CARTESIAN_POINT ( 'NONE',  ( 2.003086131649545506E-15, 29.19062499938548783, 13.33755215474603162 ) ) ;
#2809=ORIENTED_EDGE ( 'NONE', *, *, #22800, .F. ) ;
#2810=ORIENTED_EDGE ( 'NONE', *, *, #20276, .T. ) ;
#2816=DIRECTION ( 'NONE',  ( -0.000000000000000000, 1.000000000000000000, -0.000000000000000000 ) ) ;
#2817=CARTESIAN_POINT ( 'NONE',  ( -1.878215178124994722, 26.64062499938549067, 5.746835883940462963 ) ) ;
#2819=CARTESIAN_POINT ( 'NONE',  ( 4.000000000000003553, 25.45000000000000639, 8.999999999999992895 ) ) ;
#2821=CARTESIAN_POINT ( 'NONE',  ( 2.006336132164985451E-12, 39.00000000001113420, 3.500000000010202061 ) ) ;
#2831=CARTESIAN_POINT ( 'NONE',  ( -5.840899737312955864, 38.49999999999999289, 10.37254881831481512 ) ) ;
#2846=ORIENTED_EDGE ( 'NONE', *, *, #15366, .F. ) ;
#2851=CARTESIAN_POINT ( 'NONE',  ( 8.012344526598182026E-15, 28.06562499938548783, 4.662447845253954171 ) ) ;
#2860=UNCERTAINTY_MEASURE_WITH_UNIT (LENGTH_MEASURE( 1.000000000000000082E-05 ), #7555, 'distance_accuracy_value', 'NONE');
#2874=FACE_OUTER_BOUND ( 'NONE', #15489, .T. ) ;
#2878=ORIENTED_EDGE ( 'NONE', *, *, #14687, .T. ) ;
#2885=CARTESIAN_POINT ( 'NONE',  ( 3.469446951953614189E-15, 35.50000000000000711, 8.999999999999992895 ) ) ;
#2917=CARTESIAN_POINT ( 'NONE',  ( 5.112995299272250684E-15, 27.75624999877097565, 4.999999999999992006 ) ) ;
#2944=CARTESIAN_POINT ( 'NONE',  ( 3.756430356250004099, 28.81562499938548783, 11.16877607737301403 ) ) ;
#2950=CARTESIAN_POINT ( 'NONE',  ( 4.000000000000002665, 27.28749999999999787, 6.690598923241489970 ) ) ;
#2956=CARTESIAN_POINT ( 'NONE',  ( 3.756430356250004099, 26.07812499938549067, 6.831223922626973533 ) ) ;
#2960=CARTESIAN_POINT ( 'NONE',  ( 1.878215178125006934, 29.26562499938549067, 5.746835883940462963 ) ) ;
#2989=CARTESIAN_POINT ( 'NONE',  ( 3.469446951953614189E-15, 31.50000000000000000, 8.999999999999992895 ) ) ;
#2991=CARTESIAN_POINT ( 'NONE',  ( -1.878215178124999829, 27.80312499938548854, 12.25316411605951927 ) ) ;
#2997=CARTESIAN_POINT ( 'NONE',  ( -3.526711513758413297, 38.89679573513893729, 4.645898033752330569 ) ) ;
#3028=AXIS2_PLACEMENT_3D ( 'NONE', #13833, #18269, #24141 ) ;
#3070=CARTESIAN_POINT ( 'NONE',  ( -1.999999999999998224, 28.39374999877097139, 12.46410161513774639 ) ) ;
#3076=CARTESIAN_POINT ( 'NONE',  ( -3.756430356249994329, 29.11562499938548854, 11.16877607737301048 ) ) ;
#3088=CARTESIAN_POINT ( 'NONE',  ( 4.006172263299091013E-15, 28.40312499938548996, 4.662447845253954171 ) ) ;
#3090=CARTESIAN_POINT ( 'NONE',  ( 1.071796769724494558, 25.35759618943234628, 12.99999999999999467 ) ) ;
#3091=PRODUCT_CONTEXT ( 'NONE', #25153, 'mechanical' ) ;
#3093=DIRECTION ( 'NONE',  ( 0.000000000000000000, 0.000000000000000000, -1.000000000000000000 ) ) ;
#3118=CARTESIAN_POINT ( 'NONE',  ( -1.878215178124999829, 26.90312499938548640, 12.25316411605951927 ) ) ;
#3124=CARTESIAN_POINT ( 'NONE',  ( 4.000000000000005329, 26.80000000000000426, 8.999999999999992895 ) ) ;
#3130=DIRECTION ( 'NONE',  ( -1.000000000000000000, 0.000000000000000000, 0.000000000000000000 ) ) ;
#3136=EDGE_CURVE ( 'NONE', #20975, #22395, #15113, .T. ) ;
#3141=DIRECTION ( 'NONE',  ( 0.000000000000000000, 0.000000000000000000, 1.000000000000000000 ) ) ;
#3168=CARTESIAN_POINT ( 'NONE',  ( 3.469446951953614189E-15, 39.50000000000000000, 8.999999999999992895 ) ) ;
#3188=CARTESIAN_POINT ( 'NONE',  ( -3.999999999999999556, 27.45624999877097139, 11.30940107675849404 ) ) ;
#3202=CARTESIAN_POINT ( 'NONE',  ( 3.756430356250004987, 25.14062499938548356, 8.999999999999992895 ) ) ;
#3204=CARTESIAN_POINT ( 'NONE',  ( -3.999999999999996447, 25.63750000000000284, 6.690598923241487306 ) ) ;
#3205=CARTESIAN_POINT ( 'NONE',  ( 4.000000000000002665, 25.48750000000000426, 6.690598923241489970 ) ) ;
#3232=CARTESIAN_POINT ( 'NONE',  ( 1.878215178125003382, 28.02812499938548996, 5.746835883940462963 ) ) ;
#3235=VECTOR ( 'NONE', #23585, 1000.000000000000000 ) ;
#3237=CYLINDRICAL_SURFACE ( 'NONE', #9712, 0.5000000000000000000 ) ;
#3255=ORIENTED_EDGE ( 'NONE', *, *, #23050, .F. ) ;
#3256=( BOUNDED_CURVE ( )  B_SPLINE_CURVE ( 2, ( #24130, #6216, #10263, #14208, #18257, #2950, #20858, #16561, #21004 ),
 .UNSPECIFIED., .F., .F. ) 
 B_SPLINE_CURVE_WITH_KNOTS ( ( 3, 2, 2, 2, 3 ),
 ( 0.4750000000000000333, 0.4833333333333333370, 0.5000000000000000000, 0.5166666666666667185, 0.5250000000000000222 ),
 .UNSPECIFIED. ) 
 CURVE ( )  GEOMETRIC_REPRESENTATION_ITEM ( )  RATIONAL_B_SPLINE_CURVE ( ( 0.9330127018922194093, 0.9330127018922196314, 1.000000000000000000, 0.8660254037844387076, 1.000000000000000000, 0.8660254037844387076, 1.000000000000000000, 0.9330127018922194093, 0.9330127018922194093 ) ) 
 REPRESENTATION_ITEM ( '' )  );
#3283=CARTESIAN_POINT ( 'NONE',  ( -1.999999999999996669, 25.15000000000000568, 5.535898384862237620 ) ) ;
#3296=EDGE_CURVE ( 'NONE', #6423, #8768, #15495, .T. ) ;
#3314=CARTESIAN_POINT ( 'NONE',  ( 0.000000000000000000, 27.98124999877096997, 13.61880215351699874 ) ) ;
#3315=VECTOR ( 'NONE', #12743, 1000.000000000000000 ) ;
#3330=CARTESIAN_POINT ( 'NONE',  ( 3.756430356250004987, 26.49062499938548854, 8.999999999999992895 ) ) ;
#3334=CARTESIAN_POINT ( 'NONE',  ( -3.756430356249996105, 29.37812499938548427, 6.831223922626973533 ) ) ;
#3346=CARTESIAN_POINT ( 'NONE',  ( -3.526711513754876570, 31.50000000000000000, 4.145898033750337497 ) ) ;
#3365=CARTESIAN_POINT ( 'NONE',  ( 2.003086131649545506E-15, 26.94062499938549138, 13.33755215474602984 ) ) ;
#3369=AXIS2_PLACEMENT_3D ( 'NONE', #16247, #24085, #4343 ) ;
#3370=EDGE_CURVE ( 'NONE', #25139, #13400, #22582, .T. ) ;
#3375=CARTESIAN_POINT ( 'NONE',  ( 1.071796769724487675, 29.14240381056766793, 4.999999999999988454 ) ) ;
#3381=CARTESIAN_POINT ( 'NONE',  ( 5.751896526290533274, 38.59087187958030540, 7.645898033760228252 ) ) ;
#3386=FACE_OUTER_BOUND ( 'NONE', #11409, .T. ) ;
#3402=EDGE_CURVE ( 'NONE', #17275, #16647, #24435, .T. ) ;
#3403=CARTESIAN_POINT ( 'NONE',  ( 5.577813053751546416E-15, 27.81250000000000355, 4.999999999999992006 ) ) ;
#3424=ORIENTED_EDGE ( 'NONE', *, *, #12800, .F. ) ;
#3430=AXIS2_PLACEMENT_3D ( 'NONE', #5908, #13895, #20015 ) ;
#3433=ORIENTED_EDGE ( 'NONE', *, *, #22465, .T. ) ;
#3454=CARTESIAN_POINT ( 'NONE',  ( 2.000000000000005329, 28.16874999877097352, 5.535898384862238508 ) ) ;
#3470=CARTESIAN_POINT ( 'NONE',  ( 4.006172263299091013E-15, 28.17812499938548498, 13.33755215474603162 ) ) ;
#3472=CARTESIAN_POINT ( 'NONE',  ( 4.648177544792955347E-16, 25.78750000000000497, 12.99999999999999289 ) ) ;
#3473=CARTESIAN_POINT ( 'NONE',  ( 4.000000000000002665, 27.28749999999999787, 6.690598923241489970 ) ) ;
#3482=EDGE_CURVE ( 'NONE', #11943, #15750, #16792, .T. ) ;
#3493=CARTESIAN_POINT ( 'NONE',  ( -3.756430356249996549, 25.44062499938548783, 6.831223922626973533 ) ) ;
#3500=VERTEX_POINT ( 'NONE', #8669 ) ;
#3502=CARTESIAN_POINT ( 'NONE',  ( 4.006172263299091013E-15, 25.70312499938548356, 4.662447845253954171 ) ) ;
#3524=CARTESIAN_POINT ( 'NONE',  ( -5.606865722240301331, 38.73198406056108922, 7.645898033750359701 ) ) ;
#3529=ORIENTED_EDGE ( 'NONE', *, *, #23959, .F. ) ;
#3533=CARTESIAN_POINT ( 'NONE',  ( -3.169364099030547166, 38.99989214654019776, 13.49581827627000763 ) ) ;
#3535=CARTESIAN_POINT ( 'NONE',  ( 3.756430356250000546, 25.55312499938548498, 11.16877607737301226 ) ) ;
#3551=DIRECTION ( 'NONE',  ( 0.000000000000000000, 0.000000000000000000, 1.000000000000000000 ) ) ;
#3555=ORIENTED_EDGE ( 'NONE', *, *, #12503, .T. ) ;
#3579=CARTESIAN_POINT ( 'NONE',  ( 4.000000000000007105, 28.58124999877097139, 6.690598923241489970 ) ) ;
#3584=EDGE_LOOP ( 'NONE', ( #18839, #20354, #8024, #1431 ) ) ;
#3585=ORIENTED_EDGE ( 'NONE', *, *, #24328, .F. ) ;
#3590=CARTESIAN_POINT ( 'NONE',  ( 1.878215178125001605, 27.76562499938548711, 12.25316411605952283 ) ) ;
#3592=CARTESIAN_POINT ( 'NONE',  ( -1.999999999999998224, 27.55000000000000426, 12.46410161513774639 ) ) ;
#3609=VERTEX_POINT ( 'NONE', #17872 ) ;
#3612=CARTESIAN_POINT ( 'NONE',  ( 3.756430356250004987, 25.25312499938548427, 8.999999999999992895 ) ) ;
#3621=CARTESIAN_POINT ( 'NONE',  ( -3.756430356249996549, 29.52812499938548996, 8.999999999999992895 ) ) ;
#3626=( NAMED_UNIT ( * ) SI_UNIT ( $, .STERADIAN. ) SOLID_ANGLE_UNIT ( ) );
#3628=CARTESIAN_POINT ( 'NONE',  ( 4.648177544792955347E-16, 28.48750000000000071, 12.99999999999999289 ) ) ;
#3641=CARTESIAN_POINT ( 'NONE',  ( -3.756430356249996105, 29.49062499938548854, 6.831223922626973533 ) ) ;
#3643=CARTESIAN_POINT ( 'NONE',  ( 2.000000000000000000, 28.46874999877097423, 12.46410161513774817 ) ) ;
#3652=CARTESIAN_POINT ( 'NONE',  ( 4.006172263299091013E-15, 25.70312499938548356, 4.662447845253954171 ) ) ;
#3674=CYLINDRICAL_SURFACE ( 'NONE', #355, 0.5000000000000004441 ) ;
#3683=CARTESIAN_POINT ( 'NONE',  ( 0.4995657836784091477, 31.50000000000000000, 14.97916666666665897 ) ) ;
#3686=CARTESIAN_POINT ( 'NONE',  ( -4.000000000000000888, 25.71250000000000568, 11.30940107675849404 ) ) ;
#3692=DIRECTION ( 'NONE',  ( -0.000000000000000000, -1.000000000000000000, -0.000000000000000000 ) ) ;
#3697=ORIENTED_EDGE ( 'NONE', *, *, #5014, .T. ) ;
#3699=CARTESIAN_POINT ( 'NONE',  ( -3.999999999999998224, 29.66874999877097352, 8.999999999999992895 ) ) ;
#3703=CARTESIAN_POINT ( 'NONE',  ( -3.999999999999999112, 29.31250000000000000, 11.30940107675849404 ) ) ;
#3708=AXIS2_PLACEMENT_3D ( 'NONE', #15844, #23817, #4545 ) ;
#3712=CARTESIAN_POINT ( 'NONE',  ( 1.878215178124998275, 26.86562499938548854, 12.25316411605952283 ) ) ;
#3714=CARTESIAN_POINT ( 'NONE',  ( 2.000000000000005329, 26.42500000000000426, 5.535898384862238508 ) ) ;
#3717=CYLINDRICAL_SURFACE ( 'NONE', #12602, 4.000000000000000000 ) ;
#3723=CARTESIAN_POINT ( 'NONE',  ( 5.112995299272250684E-15, 26.40624999877096712, 4.999999999999992006 ) ) ;
#3728=CARTESIAN_POINT ( 'NONE',  ( 4.000000000000001776, 27.19374999877097210, 8.999999999999992895 ) ) ;
#3743=ORIENTED_EDGE ( 'NONE', *, *, #22970, .T. ) ;
#3748=CARTESIAN_POINT ( 'NONE',  ( 3.756430356250003211, 29.30312499938548498, 8.999999999999992895 ) ) ;
#3749=AXIS2_PLACEMENT_3D ( 'NONE', #7003, #19036, #17081 ) ;
#3771=ADVANCED_FACE ( 'NONE', ( #20035 ), #2138, .T. ) ;
#3777=EDGE_LOOP ( 'NONE', ( #22597, #13485, #22888, #23715 ) ) ;
#3779=ORIENTED_EDGE ( 'NONE', *, *, #17901, .T. ) ;
#3780=AXIS2_PLACEMENT_3D ( 'NONE', #4080, #1882, #9844 ) ;
#3786=CARTESIAN_POINT ( 'NONE',  ( -3.574812588380618106, 38.86762122992235646, 13.35267830710396630 ) ) ;
#3790=CIRCLE ( 'NONE', #882, 6.000000000000000000 ) ;
#3807=DIRECTION ( 'NONE',  ( 0.000000000000000000, 0.000000000000000000, -1.000000000000000000 ) ) ;
#3810=ORIENTED_EDGE ( 'NONE', *, *, #19844, .T. ) ;
#3828=CARTESIAN_POINT ( 'NONE',  ( -3.999999999999996447, 27.38124999877097210, 6.690598923241487306 ) ) ;
#3829=DIRECTION ( 'NONE',  ( 0.000000000000000000, 0.000000000000000000, -1.000000000000000000 ) ) ;
#3834=LINE ( 'NONE', #11814, #3235 ) ;
#3838=CARTESIAN_POINT ( 'NONE',  ( -2.003086131649545506E-15, 26.04062499938549280, 13.33755215474602984 ) ) ;
#3853=CARTESIAN_POINT ( 'NONE',  ( 3.756430356250003211, 28.29062499938548569, 8.999999999999992895 ) ) ;
#3854=ADVANCED_FACE ( 'NONE', ( #18101 ), #8019, .T. ) ;
#3857=CARTESIAN_POINT ( 'NONE',  ( 2.000000000000000000, 26.72500000000000497, 12.46410161513774817 ) ) ;
#3885=CARTESIAN_POINT ( 'NONE',  ( 1.878215178125001605, 26.41562499938548925, 12.25316411605952283 ) ) ;
#3896=CARTESIAN_POINT ( 'NONE',  ( -8.366719580627318441E-15, 29.55624999877097281, 4.999999999999992006 ) ) ;
#3901=ORIENTED_EDGE ( 'NONE', *, *, #21565, .T. ) ;
#3903=CARTESIAN_POINT ( 'NONE',  ( 5.201626763664007669, 38.97563867572937824, 7.138217499902562935 ) ) ;
#3909=FACE_BOUND ( 'NONE', #19795, .T. ) ;
#3918=VERTEX_POINT ( 'NONE', #10207 ) ;
#3921=CARTESIAN_POINT ( 'NONE',  ( 6.009258394948636914E-15, 26.60312499938547859, 4.662447845253954171 ) ) ;
#3941=ORIENTED_EDGE ( 'NONE', *, *, #18233, .F. ) ;
#3944=ORIENTED_EDGE ( 'NONE', *, *, #4797, .T. ) ;
#3962=SHAPE_DEFINITION_REPRESENTATION ( #16341, #22515 ) ;
#3966=CARTESIAN_POINT ( 'NONE',  ( 1.071796769724497222, 28.05759618943234202, 12.99999999999998757 ) ) ;
#3967=EDGE_LOOP ( 'NONE', ( #16984, #17177, #13654, #12427 ) ) ;
#3969=CARTESIAN_POINT ( 'NONE',  ( -3.756430356249997882, 25.92812499938548854, 8.999999999999992895 ) ) ;
#3978=CARTESIAN_POINT ( 'NONE',  ( 5.577813053751546416E-15, 25.95624999877097139, 4.999999999999992006 ) ) ;
#3982=CARTESIAN_POINT ( 'NONE',  ( 6.009258394948636914E-15, 27.50312499938549138, 4.662447845253954171 ) ) ;
#3984=CARTESIAN_POINT ( 'NONE',  ( 2.000000000000005329, 28.22500000000000497, 5.535898384862238508 ) ) ;
#3994=CARTESIAN_POINT ( 'NONE',  ( -5.840899737312982509, 31.50000000000000000, 7.627451181685283466 ) ) ;
#3999=CARTESIAN_POINT ( 'NONE',  ( 1.878215178125003382, 26.67812499938548854, 5.746835883940462963 ) ) ;
#4009=CARTESIAN_POINT ( 'NONE',  ( -3.756430356249996105, 26.67812499938548854, 6.831223922626973533 ) ) ;
#4025=ADVANCED_FACE ( 'NONE', ( #418 ), #5770, .T. ) ;
#4028=EDGE_LOOP ( 'NONE', ( #14703, #25556, #5591, #20296 ) ) ;
#4032=CARTESIAN_POINT ( 'NONE',  ( 4.000000000000002665, 28.50624999877097210, 11.30940107675849760 ) ) ;
#4040=CARTESIAN_POINT ( 'NONE',  ( -3.118462878979592734, 38.97860908142764913, 13.55684613422404006 ) ) ;
#4041=CARTESIAN_POINT ( 'NONE',  ( -3.756430356249998326, 27.20312499938549067, 11.16877607737301226 ) ) ;
#4050=CARTESIAN_POINT ( 'NONE',  ( 1.580380365229604700E-14, 27.58750000000000213, 12.99999999999999289 ) ) ;
#4054=FACE_OUTER_BOUND ( 'NONE', #11297, .T. ) ;
#4062=ORIENTED_EDGE ( 'NONE', *, *, #3370, .F. ) ;
#4075=CYLINDRICAL_SURFACE ( 'NONE', #865, 4.000000000000000000 ) ;
#4080=CARTESIAN_POINT ( 'NONE',  ( 3.469446951953614189E-15, 35.50000000000000711, 8.999999999999992895 ) ) ;
#4085=CARTESIAN_POINT ( 'NONE',  ( 3.756430356250004987, 26.60312499938548569, 8.999999999999992895 ) ) ;
#4100=CARTESIAN_POINT ( 'NONE',  ( 3.756430356250002323, 29.60312499938548925, 11.16877607737301403 ) ) ;
#4103=CARTESIAN_POINT ( 'NONE',  ( -3.999999999999996447, 28.33750000000000568, 6.690598923241487306 ) ) ;
#4111=CARTESIAN_POINT ( 'NONE',  ( -0.4972522109372425891, 38.55547752541761497, 3.076310858750954225 ) ) ;
#4121=CARTESIAN_POINT ( 'NONE',  ( 3.756430356250004987, 26.60312499938548569, 8.999999999999992895 ) ) ;
#4130=CARTESIAN_POINT ( 'NONE',  ( -1.878215178124998275, 27.24062499938548854, 12.25316411605951927 ) ) ;
#4142=LINE ( 'NONE', #13968, #1746 ) ;
#4154=CARTESIAN_POINT ( 'NONE',  ( -1.999999999999996669, 26.20000000000000639, 12.46410161513774639 ) ) ;
#4160=FACE_OUTER_BOUND ( 'NONE', #22009, .T. ) ;
#4170=CARTESIAN_POINT ( 'NONE',  ( 6.009258394948636914E-15, 27.95312499938548356, 4.662447845253954171 ) ) ;
#4177=DIRECTION ( 'NONE',  ( -0.000000000000000000, -1.000000000000000000, -0.000000000000000000 ) ) ;
#4178=FACE_OUTER_BOUND ( 'NONE', #6188, .T. ) ;
#4225=CARTESIAN_POINT ( 'NONE',  ( 2.000000000000007105, 29.51874999877097139, 5.535898384862238508 ) ) ;
#4227=DIRECTION ( 'NONE',  ( 0.000000000000000000, 0.000000000000000000, -1.000000000000000000 ) ) ;
#4239=CARTESIAN_POINT ( 'NONE',  ( 3.469446951953614189E-15, 39.50000000000000000, 8.999999999999992895 ) ) ;
#4241=CARTESIAN_POINT ( 'NONE',  ( 4.000000000000002665, 28.56249999999999645, 11.30940107675849760 ) ) ;
#4247=CIRCLE ( 'NONE', #19274, 0.5000000000000004441 ) ;
#4257=CARTESIAN_POINT ( 'NONE',  ( 5.206848532682268882, 39.00010698140258825, 10.77302451745546286 ) ) ;
#4261=CARTESIAN_POINT ( 'NONE',  ( -3.756430356249996549, 27.76562499938549422, 11.16877607737301048 ) ) ;
#4267=FACE_OUTER_BOUND ( 'NONE', #415, .T. ) ;
#4270=VERTEX_POINT ( 'NONE', #23540 ) ;
#4272=CIRCLE ( 'NONE', #3028, 0.5000000000000000000 ) ;
#4273=CARTESIAN_POINT ( 'NONE',  ( -3.756430356249994773, 28.96562499938548640, 8.999999999999992895 ) ) ;
#4281=DIRECTION ( 'NONE',  ( 0.000000000000000000, -1.000000000000000000, 0.000000000000000000 ) ) ;
#4289=DIRECTION ( 'NONE',  ( 0.000000000000000000, 0.000000000000000000, -1.000000000000000000 ) ) ;
#4301=CARTESIAN_POINT ( 'NONE',  ( 3.110308778861319290, 38.49999999999999289, 3.869115154270335477 ) ) ;
#4308=CARTESIAN_POINT ( 'NONE',  ( -3.756430356249996105, 25.89062499938548356, 6.831223922626973533 ) ) ;
#4310=CARTESIAN_POINT ( 'NONE',  ( -1.999999999999998224, 28.90000000000000924, 12.46410161513774639 ) ) ;
#4335=EDGE_CURVE ( 'NONE', #3918, #15046, #7065, .T. ) ;
#4341=CARTESIAN_POINT ( 'NONE',  ( 2.000000000000003553, 25.97500000000000497, 5.535898384862238508 ) ) ;
#4343=DIRECTION ( 'NONE',  ( 5.329070518200752183E-15, 0.000000000000000000, 1.000000000000000000 ) ) ;
#4344=DIRECTION ( 'NONE',  ( 0.000000000000000000, 0.000000000000000000, -1.000000000000000000 ) ) ;
#4350=CARTESIAN_POINT ( 'NONE',  ( -1.022599059854450137E-14, 29.16250000000000497, 4.999999999999992006 ) ) ;
#4353=ORIENTED_EDGE ( 'NONE', *, *, #22461, .F. ) ;
#4354=CARTESIAN_POINT ( 'NONE',  ( 3.756430356250002323, 27.91562499938548925, 11.16877607737301226 ) ) ;
#4359=CARTESIAN_POINT ( 'NONE',  ( -3.999999999999996447, 28.37500000000000355, 8.999999999999992895 ) ) ;
#4369=CYLINDRICAL_SURFACE ( 'NONE', #11246, 4.000000000000000000 ) ;
#4371=B_SPLINE_CURVE_WITH_KNOTS ( 'NONE', 3,
 ( #600, #4111, #14334, #18370, #10639, #2408, #22299, #4374, #12473, #12352 ),
 .UNSPECIFIED., .F., .F.,
 ( 4, 2, 2, 2, 4 ),
 ( 2.789812635309770584E-07, 0.0002324414413947193921, 0.0004646039015259078100, 0.0006967663616570962280, 0.0009289288217882846459 ),
 .UNSPECIFIED. ) ;
#4374=CARTESIAN_POINT ( 'NONE',  ( -0.1550712154452952851, 38.97879272568130204, 3.480616423035832518 ) ) ;
#4375=CARTESIAN_POINT ( 'NONE',  ( -1.999999999999994893, 25.54374999877097352, 5.535898384862237620 ) ) ;
#4378=CARTESIAN_POINT ( 'NONE',  ( -0.4995657836784015426, 34.50000000000000000, 3.020833333333324600 ) ) ;
#4382=CARTESIAN_POINT ( 'NONE',  ( 3.756430356250006319, 27.09062499938548640, 6.831223922626973533 ) ) ;
#4386=CARTESIAN_POINT ( 'NONE',  ( 3.611975211414842679, 38.84312993071436892, 4.645898033752072998 ) ) ;
#4392=CARTESIAN_POINT ( 'NONE',  ( -3.756430356249996105, 27.65312499938548996, 11.16877607737301226 ) ) ;
#4422=VERTEX_POINT ( 'NONE', #13860 ) ;
#4425=ORIENTED_EDGE ( 'NONE', *, *, #25507, .F. ) ;
#4435=CARTESIAN_POINT ( 'NONE',  ( 3.469446951953614189E-15, 35.50000000000000711, 4.999999999999992006 ) ) ;
#4439=DIRECTION ( 'NONE',  ( 0.000000000000000000, 0.000000000000000000, 1.000000000000000000 ) ) ;
#4442=CARTESIAN_POINT ( 'NONE',  ( -4.000000000000000000, 27.47500000000000142, 8.999999999999992895 ) ) ;
#4445=ADVANCED_BREP_SHAPE_REPRESENTATION ( '', ( #5394, #21036 ), #21481 ) ;
#4465=FACE_OUTER_BOUND ( 'NONE', #1443, .T. ) ;
#4476=CARTESIAN_POINT ( 'NONE',  ( 3.756430356250002323, 27.46562499938548640, 11.16877607737301226 ) ) ;
#4490=PLANE ( 'NONE',  #9233 ) ;
#4499=CARTESIAN_POINT ( 'NONE',  ( 4.000000000000003553, 25.39374999877097494, 8.999999999999992895 ) ) ;
#4502=CARTESIAN_POINT ( 'NONE',  ( 5.532151103383248447, 38.49999999999999289, 11.32277940608563149 ) ) ;
#4506=CARTESIAN_POINT ( 'NONE',  ( -3.756430356249997882, 28.66562499938548925, 11.16877607737301048 ) ) ;
#4515=CARTESIAN_POINT ( 'NONE',  ( 6.009258394948636914E-15, 27.50312499938549138, 4.662447845253954171 ) ) ;
#4517=CARTESIAN_POINT ( 'NONE',  ( 4.000000000000000888, 26.31250000000000711, 11.30940107675849760 ) ) ;
#4537=CARTESIAN_POINT ( 'NONE',  ( -3.999999999999996447, 25.58124999877097139, 6.690598923241487306 ) ) ;
#4545=DIRECTION ( 'NONE',  ( 0.000000000000000000, 0.000000000000000000, 1.000000000000000000 ) ) ;
#4552=CARTESIAN_POINT ( 'NONE',  ( 1.878215178125001605, 26.07812499938549067, 12.25316411605952283 ) ) ;
#4555=( BOUNDED_CURVE ( )  B_SPLINE_CURVE ( 2, ( #2450, #8721, #22852, #4537, #633, #884, #10553, #8868, #12266 ),
 .UNSPECIFIED., .F., .F. ) 
 B_SPLINE_CURVE_WITH_KNOTS ( ( 3, 2, 2, 2, 3 ),
 ( 0.02500000000000000486, 0.03333333333333333287, 0.05000000000000000278, 0.06666666666666666574, 0.07500000000000001110 ),
 .UNSPECIFIED. ) 
 CURVE ( )  GEOMETRIC_REPRESENTATION_ITEM ( )  RATIONAL_B_SPLINE_CURVE ( ( 0.9330127018922194093, 0.9330127018922194093, 1.000000000000000000, 0.8660254037844387076, 1.000000000000000000, 0.8660254037844387076, 1.000000000000000000, 0.9330127018922191873, 0.9330127018922192983 ) ) 
 REPRESENTATION_ITEM ( '' )  );
#4577=CARTESIAN_POINT ( 'NONE',  ( 3.469446951953614189E-15, 39.50000000000000000, 8.999999999999992895 ) ) ;
#4594=DIRECTION ( 'NONE',  ( -0.000000000000000000, -1.000000000000000000, -0.000000000000000000 ) ) ;
#4597=CIRCLE ( 'NONE', #16727, 6.000000000000000000 ) ;
#4606=AXIS2_PLACEMENT_3D ( 'NONE', #23191, #25164, #9339 ) ;
#4609=VERTEX_POINT ( 'NONE', #8493 ) ;
#4610=CARTESIAN_POINT ( 'NONE',  ( -3.756430356249997882, 27.72812499938548569, 8.999999999999992895 ) ) ;
#4615=ORIENTED_EDGE ( 'NONE', *, *, #25156, .F. ) ;
#4617=EDGE_LOOP ( 'NONE', ( #12667, #23957, #3433, #6003 ) ) ;
#4622=DIRECTION ( 'NONE',  ( 0.000000000000000000, 1.000000000000000000, -0.000000000000000000 ) ) ;
#4629=CARTESIAN_POINT ( 'NONE',  ( -3.999999999999996447, 26.53750000000000497, 6.690598923241487306 ) ) ;
#4630=CARTESIAN_POINT ( 'NONE',  ( -1.999999999999996669, 29.35000000000000853, 12.46410161513774639 ) ) ;
#4640=AXIS2_PLACEMENT_3D ( 'NONE', #3346, #19543, #13431 ) ;
#4644=CARTESIAN_POINT ( 'NONE',  ( 5.201400854508229088, 38.97868814324866094, 10.85315172130059480 ) ) ;
#4648=CARTESIAN_POINT ( 'NONE',  ( 3.756430356250004987, 29.75312499938549138, 8.999999999999992895 ) ) ;
#4656=CARTESIAN_POINT ( 'NONE',  ( 3.756430356250006319, 28.77812499938548640, 6.831223922626973533 ) ) ;
#4660=CARTESIAN_POINT ( 'NONE',  ( -3.756430356249996549, 26.71562499938548996, 8.999999999999992895 ) ) ;
#4674=CARTESIAN_POINT ( 'NONE',  ( -5.734022625014068453, 38.61087488181074434, 10.34268409280109502 ) ) ;
#4687=CYLINDRICAL_SURFACE ( 'NONE', #11242, 0.5000000000000004441 ) ;
#4689=AXIS2_PLACEMENT_3D ( 'NONE', #5247, #1331, #17673 ) ;
#4723=ORIENTED_EDGE ( 'NONE', *, *, #7399, .F. ) ;
#4730=VERTEX_POINT ( 'NONE', #524 ) ;
#4747=LINE ( 'NONE', #18862, #19222 ) ;
#4759=CARTESIAN_POINT ( 'NONE',  ( -1.878215178124996498, 29.00312499938548783, 5.746835883940462963 ) ) ;
#4767=CARTESIAN_POINT ( 'NONE',  ( 3.526711513754818395, 29.50000000000000000, 4.645898033750289535 ) ) ;
#4769=EDGE_CURVE ( 'NONE', #10104, #4609, #21158, .T. ) ;
#4774=EDGE_CURVE ( 'NONE', #1139, #25560, #14325, .T. ) ;
#4778=CARTESIAN_POINT ( 'NONE',  ( 4.000000000000002665, 26.33124999877097494, 6.690598923241489970 ) ) ;
#4784=CARTESIAN_POINT ( 'NONE',  ( -1.878215178124996498, 29.45312499938548711, 5.746835883940462963 ) ) ;
#4790=ORIENTED_EDGE ( 'NONE', *, *, #21668, .F. ) ;
#4792=CARTESIAN_POINT ( 'NONE',  ( 3.756430356250002323, 29.60312499938548925, 11.16877607737301226 ) ) ;
#4793=CARTESIAN_POINT ( 'NONE',  ( 1.878215178125003382, 26.11562499938548854, 5.746835883940462963 ) ) ;
#4795=CARTESIAN_POINT ( 'NONE',  ( 3.756430356250003211, 26.94062499938548783, 8.999999999999992895 ) ) ;
#4796=CARTESIAN_POINT ( 'NONE',  ( -1.999999999999994893, 28.75000000000000355, 5.535898384862237620 ) ) ;
#4797=EDGE_CURVE ( 'NONE', #22637, #13892, #21838, .T. ) ;
#4822=CARTESIAN_POINT ( 'NONE',  ( 4.006172263299091013E-15, 27.16562499938548569, 4.662447845253954171 ) ) ;
#4824=EDGE_CURVE ( 'NONE', #15750, #15689, #19308, .T. ) ;
#4836=ADVANCED_FACE ( 'NONE', ( #17749 ), #11590, .T. ) ;
#4842=ORIENTED_EDGE ( 'NONE', *, *, #22461, .T. ) ;
#4850=VERTEX_POINT ( 'NONE', #11858 ) ;
#4857=FACE_OUTER_BOUND ( 'NONE', #4617, .T. ) ;
#4867=CARTESIAN_POINT ( 'NONE',  ( -1.071796769724487453, 25.13259618943234486, 4.999999999999992006 ) ) ;
#4868=CARTESIAN_POINT ( 'NONE',  ( 3.526711513754818395, 29.50000000000000000, 4.145898033750289535 ) ) ;
#4872=CARTESIAN_POINT ( 'NONE',  ( -1.878215178124996498, 27.65312499938548996, 5.746835883940462963 ) ) ;
#4873=EDGE_CURVE ( 'NONE', #23529, #8768, #16019, .T. ) ;
#4874=ORIENTED_EDGE ( 'NONE', *, *, #17793, .T. ) ;
#4893=VERTEX_POINT ( 'NONE', #21388 ) ;
#4895=CARTESIAN_POINT ( 'NONE',  ( 6.009258394948636914E-15, 26.40624999877097423, 4.381197846482986158 ) ) ;
#4901=CARTESIAN_POINT ( 'NONE',  ( 3.756430356250004099, 29.34062499938548640, 6.831223922626973533 ) ) ;
#4909=CARTESIAN_POINT ( 'NONE',  ( -2.003086131649545506E-15, 26.82812499938549067, 13.33755215474603162 ) ) ;
#4911=CARTESIAN_POINT ( 'NONE',  ( 4.000000000000002665, 25.86250000000000071, 11.30940107675849760 ) ) ;
#4930=FACE_OUTER_BOUND ( 'NONE', #6315, .T. ) ;
#4934=ORIENTED_EDGE ( 'NONE', *, *, #2469, .F. ) ;
#4941=CARTESIAN_POINT ( 'NONE',  ( 3.756430356250002323, 27.91562499938548925, 11.16877607737301226 ) ) ;
#4972=AXIS2_PLACEMENT_3D ( 'NONE', #482, #24404, #14855 ) ;
#5014=EDGE_CURVE ( 'NONE', #17574, #22373, #2481, .T. ) ;
#5020=EDGE_CURVE ( 'NONE', #2753, #19084, #10301, .T. ) ;
#5021=VECTOR ( 'NONE', #810, 1000.000000000000000 ) ;
#5029=CARTESIAN_POINT ( 'NONE',  ( 8.012344526598182026E-15, 26.85624999877096997, 4.381197846482986158 ) ) ;
#5045=CARTESIAN_POINT ( 'NONE',  ( -1.878215178124994722, 29.34062499938548640, 5.746835883940462963 ) ) ;
#5046=CARTESIAN_POINT ( 'NONE',  ( 3.756430356250003211, 26.04062499938548925, 8.999999999999992895 ) ) ;
#5048=DIRECTION ( 'NONE',  ( 0.000000000000000000, 0.000000000000000000, 1.000000000000000000 ) ) ;
#5049=CARTESIAN_POINT ( 'NONE',  ( 4.006172263299091013E-15, 28.17812499938548498, 13.33755215474602984 ) ) ;
#5084=CARTESIAN_POINT ( 'NONE',  ( 3.756430356250003211, 28.85312499938548569, 8.999999999999992895 ) ) ;
#5087=EDGE_CURVE ( 'NONE', #22637, #22373, #16146, .T. ) ;
#5089=EDGE_CURVE ( 'NONE', #19084, #22278, #7806, .T. ) ;
#5107=DIRECTION ( 'NONE',  ( 0.000000000000000000, 0.000000000000000000, 1.000000000000000000 ) ) ;
#5109=CARTESIAN_POINT ( 'NONE',  ( -5.242581649506213637, 39.00274862415032118, 7.344859984781824558 ) ) ;
#5132=CARTESIAN_POINT ( 'NONE',  ( 5.532151103383234236, 34.50000000000000000, 6.677220593914319657 ) ) ;
#5135=CARTESIAN_POINT ( 'NONE',  ( -1.071796769724489895, 29.76115380933864429, 12.99999999999999289 ) ) ;
#5167=EDGE_CURVE ( 'NONE', #12364, #22278, #194, .T. ) ;
#5168=CARTESIAN_POINT ( 'NONE',  ( -1.999999999999996669, 27.49374999877097636, 12.46410161513774639 ) ) ;
#5185=CARTESIAN_POINT ( 'NONE',  ( -3.999999999999996447, 25.22500000000000497, 8.999999999999992895 ) ) ;
#5190=CARTESIAN_POINT ( 'NONE',  ( -1.999999999999994893, 26.89374999877097849, 5.535898384862237620 ) ) ;
#5203=CARTESIAN_POINT ( 'NONE',  ( 5.840899737312970963, 34.50000000000000000, 7.627451181685208859 ) ) ;
#5212=CARTESIAN_POINT ( 'NONE',  ( 1.878215178125008489, 28.92812499938549209, 5.746835883940462963 ) ) ;
#5216=CARTESIAN_POINT ( 'NONE',  ( 4.000000000000000888, 28.63750000000000639, 6.690598923241489970 ) ) ;
#5219=DIRECTION ( 'NONE',  ( 0.000000000000000000, 0.000000000000000000, 1.000000000000000000 ) ) ;
#5220=CARTESIAN_POINT ( 'NONE',  ( 7.901901826148023498E-15, 26.23750000000000426, 12.99999999999999112 ) ) ;
#5237=ORIENTED_EDGE ( 'NONE', *, *, #7530, .T. ) ;
#5246=CARTESIAN_POINT ( 'NONE',  ( 3.469446951953614189E-15, 38.49999999999999289, 8.999999999999992895 ) ) ;
#5247=CARTESIAN_POINT ( 'NONE',  ( 3.469446951953614189E-15, 39.50000000000000000, 8.999999999999992895 ) ) ;
#5261=ORIENTED_EDGE ( 'NONE', *, *, #12763, .F. ) ;
#5269=EDGE_LOOP ( 'NONE', ( #15348, #17520, #22173, #9888, #19145 ) ) ;
#5283=CARTESIAN_POINT ( 'NONE',  ( 6.009258394948636914E-15, 28.20624999877096784, 4.381197846482986158 ) ) ;
#5293=DIRECTION ( 'NONE',  ( 0.000000000000000000, -1.000000000000000000, 0.000000000000000000 ) ) ;
#5296=CARTESIAN_POINT ( 'NONE',  ( -1.878215178124998275, 29.49062499938548854, 12.25316411605951927 ) ) ;
#5297=CARTESIAN_POINT ( 'NONE',  ( -1.878215178124996498, 26.19062499938548783, 5.746835883940462963 ) ) ;
#5299=CARTESIAN_POINT ( 'NONE',  ( 3.469446951953614189E-15, 31.50000000000000000, 8.999999999999992895 ) ) ;
#5300=CARTESIAN_POINT ( 'NONE',  ( 3.756430356250002323, 29.60312499938548925, 11.16877607737301226 ) ) ;
#5302=CARTESIAN_POINT ( 'NONE',  ( 4.000000000000005329, 25.41250000000000497, 11.30940107675849760 ) ) ;
#5328=CARTESIAN_POINT ( 'NONE',  ( -3.756430356249996549, 27.27812499938548996, 8.999999999999992895 ) ) ;
#5340=DIRECTION ( 'NONE',  ( -0.000000000000000000, 1.000000000000000000, 0.000000000000000000 ) ) ;
#5343=CARTESIAN_POINT ( 'NONE',  ( 5.797192864167126203, 38.54534174146481718, 7.639664215341221976 ) ) ;
#5347=DIRECTION ( 'NONE',  ( 0.000000000000000000, 0.000000000000000000, 1.000000000000000000 ) ) ;
#5360=VECTOR ( 'NONE', #21334, 1000.000000000000114 ) ;
#5361=CARTESIAN_POINT ( 'NONE',  ( -1.999999999999994893, 27.85000000000000497, 5.535898384862237620 ) ) ;
#5367=DIRECTION ( 'NONE',  ( 0.000000000000000000, -1.000000000000000000, 0.000000000000000000 ) ) ;
#5370=VECTOR ( 'NONE', #13168, 1000.000000000000114 ) ;
#5373=DIRECTION ( 'NONE',  ( 0.000000000000000000, 0.000000000000000000, 1.000000000000000000 ) ) ;
#5375=ADVANCED_FACE ( 'NONE', ( #19602 ), #20179, .T. ) ;
#5382=VERTEX_POINT ( 'NONE', #22927 ) ;
#5394=MANIFOLD_SOLID_BREP ( 'Cavity1', #10872 ) ;
#5400=( BOUNDED_CURVE ( )  B_SPLINE_CURVE ( 2, ( #23965, #6046, #16244, #14029, #12045, #22260, #4341, #19779, #10334 ),
 .UNSPECIFIED., .F., .F. ) 
 B_SPLINE_CURVE_WITH_KNOTS ( ( 3, 2, 2, 2, 3 ),
 ( 0.1749999999999999889, 0.1833333333333333204, 0.2000000000000000111, 0.2166666666666666741, 0.2250000000000000056 ),
 .UNSPECIFIED. ) 
 CURVE ( )  GEOMETRIC_REPRESENTATION_ITEM ( )  RATIONAL_B_SPLINE_CURVE ( ( 0.9330127018922194093, 0.9330127018922194093, 1.000000000000000000, 0.8660254037844387076, 1.000000000000000000, 0.8660254037844387076, 1.000000000000000000, 0.9330127018922194093, 0.9330127018922194093 ) ) 
 REPRESENTATION_ITEM ( '' )  );
#5407=CARTESIAN_POINT ( 'NONE',  ( 4.081770351527290718E-15, 39.50000000000000000, 13.99999999999999289 ) ) ;
#5411=CARTESIAN_POINT ( 'NONE',  ( -3.999999999999996447, 28.80624999877096926, 11.30940107675849404 ) ) ;
#5427=CARTESIAN_POINT ( 'NONE',  ( -3.756430356249996549, 28.92812499938548854, 6.831223922626973533 ) ) ;
#5430=CARTESIAN_POINT ( 'NONE',  ( 2.000000000000007105, 26.87500000000001066, 5.535898384862238508 ) ) ;
#5437=LINE ( 'NONE', #5690, #21666 ) ;
#5459=CARTESIAN_POINT ( 'NONE',  ( 0.000000000000000000, 25.92812499938548854, 13.33755215474602984 ) ) ;
#5523=ORIENTED_EDGE ( 'NONE', *, *, #10900, .T. ) ;
#5534=CARTESIAN_POINT ( 'NONE',  ( 1.071796769724491671, 29.40759618943233633, 12.99999999999999467 ) ) ;
#5547=CARTESIAN_POINT ( 'NONE',  ( 2.000000000000000000, 28.46874999877097423, 12.46410161513774817 ) ) ;
#5558=FACE_OUTER_BOUND ( 'NONE', #6328, .T. ) ;
#5559=ORIENTED_EDGE ( 'NONE', *, *, #12177, .T. ) ;
#5560=CARTESIAN_POINT ( 'NONE',  ( 0.1550712154453031122, 38.97879272568130204, 14.51938357696415416 ) ) ;
#5562=CARTESIAN_POINT ( 'NONE',  ( -3.756430356249997882, 28.10312499938548569, 11.16877607737301048 ) ) ;
#5563=FACE_OUTER_BOUND ( 'NONE', #10420, .T. ) ;
#5564=CARTESIAN_POINT ( 'NONE',  ( -1.999999999999998224, 27.10000000000000497, 12.46410161513774639 ) ) ;
#5567=AXIS2_PLACEMENT_3D ( 'NONE', #458, #24384, #14448 ) ;
#5580=DIRECTION ( 'NONE',  ( 0.000000000000000000, 0.000000000000000000, 1.000000000000000000 ) ) ;
#5591=ORIENTED_EDGE ( 'NONE', *, *, #6167, .T. ) ;
#5594=CARTESIAN_POINT ( 'NONE',  ( -1.878215178124998275, 25.44062499938549138, 12.25316411605951927 ) ) ;
#5607=CARTESIAN_POINT ( 'NONE',  ( 5.840899737312971851, 38.49999999999999289, 7.627451181685208859 ) ) ;
#5611=CARTESIAN_POINT ( 'NONE',  ( 3.884165915710650729, 38.55544002051693298, 13.50011709117523218 ) ) ;
#5653=ORIENTED_EDGE ( 'NONE', *, *, #7234, .T. ) ;
#5670=CARTESIAN_POINT ( 'NONE',  ( 2.000000000000000000, 29.81874999877097210, 12.46410161513774817 ) ) ;
#5671=ORIENTED_EDGE ( 'NONE', *, *, #1035, .T. ) ;
#5677=CARTESIAN_POINT ( 'NONE',  ( 7.901901826148023498E-15, 27.53124999877097068, 12.99999999999999112 ) ) ;
#5681=CARTESIAN_POINT ( 'NONE',  ( -3.756430356249994773, 28.96562499938548640, 8.999999999999992895 ) ) ;
#5683=CARTESIAN_POINT ( 'NONE',  ( -3.999999999999994671, 27.88750000000000639, 6.690598923241487306 ) ) ;
#5690=CARTESIAN_POINT ( 'NONE',  ( 3.110308778861319734, 34.50000000000000000, 3.869115154270335477 ) ) ;
#5695=CARTESIAN_POINT ( 'NONE',  ( 2.000000000000000000, 27.11874999877097281, 12.46410161513774817 ) ) ;
#5701=CARTESIAN_POINT ( 'NONE',  ( 3.756430356250003211, 25.70312499938548356, 8.999999999999992895 ) ) ;
#5709=DIRECTION ( 'NONE',  ( 0.000000000000000000, -1.000000000000000000, 0.000000000000000000 ) ) ;
#5710=CARTESIAN_POINT ( 'NONE',  ( 0.000000000000000000, 29.64062499938549422, 13.33755215474602984 ) ) ;
#5714=CARTESIAN_POINT ( 'NONE',  ( 1.487416814333745711E-14, 28.43124999877096926, 12.99999999999999289 ) ) ;
#5728=CARTESIAN_POINT ( 'NONE',  ( -3.999999999999996447, 26.08750000000000213, 6.690598923241487306 ) ) ;
#5729=CARTESIAN_POINT ( 'NONE',  ( 3.469446951953614189E-15, 31.50000000000000000, 8.999999999999992895 ) ) ;
#5730=VERTEX_POINT ( 'NONE', #22714 ) ;
#5732=CARTESIAN_POINT ( 'NONE',  ( -5.239945491911981890, 38.87560126879805722, 6.955677371495904815 ) ) ;
#5733=CARTESIAN_POINT ( 'NONE',  ( 4.000000000000007105, 28.58124999877097139, 6.690598923241489970 ) ) ;
#5741=CARTESIAN_POINT ( 'NONE',  ( -3.057059652155495133, 38.61000136877623135, 14.03455380423570809 ) ) ;
#5758=CARTESIAN_POINT ( 'NONE',  ( 3.878215178125001827, 25.07031249969274711, 8.999999999999992895 ) ) ;
#5759=ORIENTED_EDGE ( 'NONE', *, *, #18309, .T. ) ;
#5770=CYLINDRICAL_SURFACE ( 'NONE', #3430, 4.000000000000000000 ) ;
#5781=AXIS2_PLACEMENT_3D ( 'NONE', #21052, #19198, #3130 ) ;
#5782=EDGE_CURVE ( 'NONE', #18497, #9321, #10853, .T. ) ;
#5789=CARTESIAN_POINT ( 'NONE',  ( 6.009258394948636914E-15, 29.55624999877097636, 4.381197846482986158 ) ) ;
#5795=CARTESIAN_POINT ( 'NONE',  ( 1.859271017917182139E-15, 29.38750000000000639, 12.99999999999999289 ) ) ;
#5801=CARTESIAN_POINT ( 'NONE',  ( 4.000000000000005329, 25.03750000000000497, 6.690598923241489970 ) ) ;
#5805=CARTESIAN_POINT ( 'NONE',  ( 3.110308778861319290, 38.49999999999999289, 3.869115154270335477 ) ) ;
#5807=CARTESIAN_POINT ( 'NONE',  ( 3.756430356250004099, 26.90312499938548996, 11.16877607737301403 ) ) ;
#5810=CARTESIAN_POINT ( 'NONE',  ( -3.999999999999999556, 27.43750000000001066, 6.690598923241487306 ) ) ;
#5817=CARTESIAN_POINT ( 'NONE',  ( -3.918623196469518177, 38.49999999999999289, 4.456389954662586028 ) ) ;
#5823=CARTESIAN_POINT ( 'NONE',  ( -8.366719580627318441E-15, 29.55624999877097636, 4.999999999999992006 ) ) ;
#5829=CARTESIAN_POINT ( 'NONE',  ( -3.756430356249997882, 25.92812499938548854, 8.999999999999992895 ) ) ;
#5839=ADVANCED_FACE ( 'NONE', ( #5563 ), #21392, .T. ) ;
#5840=CARTESIAN_POINT ( 'NONE',  ( -2.003086131649545506E-15, 26.37812499938548427, 13.33755215474602984 ) ) ;
#5843=AXIS2_PLACEMENT_3D ( 'NONE', #3168, #18732, #23057 ) ;
#5847=CARTESIAN_POINT ( 'NONE',  ( -1.071796769724485232, 28.22634618820330132, 4.999999999999992006 ) ) ;
#5848=CARTESIAN_POINT ( 'NONE',  ( 3.959305671612554781E-15, 35.50000000000000711, 12.99999999999999289 ) ) ;
#5851=CARTESIAN_POINT ( 'NONE',  ( 1.071796769724490561, 29.53615380933863577, 4.999999999999988454 ) ) ;
#5852=CARTESIAN_POINT ( 'NONE',  ( 5.706339097770919189, 29.50000000000000000, 7.645898033750285983 ) ) ;
#5858=CARTESIAN_POINT ( 'NONE',  ( 5.485456488530129349, 38.54977203910393513, 6.694575048425325470 ) ) ;
#5865=CARTESIAN_POINT ( 'NONE',  ( 4.000000000000003553, 26.74374999877097281, 8.999999999999992895 ) ) ;
#5871=VERTEX_POINT ( 'NONE', #3472 ) ;
#5880=CARTESIAN_POINT ( 'NONE',  ( -3.756430356249996105, 27.57812499938548356, 6.831223922626973533 ) ) ;
#5892=CARTESIAN_POINT ( 'NONE',  ( 5.577813053751546416E-15, 27.81250000000000355, 4.999999999999992006 ) ) ;
#5896=CARTESIAN_POINT ( 'NONE',  ( 4.000000000000005329, 28.09374999877097778, 8.999999999999992895 ) ) ;
#5899=CARTESIAN_POINT ( 'NONE',  ( -1.071796769724486564, 27.11740381056766935, 12.99999999999999467 ) ) ;
#5908=CARTESIAN_POINT ( 'NONE',  ( 3.469446951953614189E-15, 35.50000000000000711, 8.999999999999992895 ) ) ;
#5921=DIRECTION ( 'NONE',  ( -0.000000000000000000, -1.000000000000000000, -0.000000000000000000 ) ) ;
#5930=CARTESIAN_POINT ( 'NONE',  ( 6.009258394948636914E-15, 26.26562499938548356, 4.662447845253954171 ) ) ;
#5933=ORIENTED_EDGE ( 'NONE', *, *, #14498, .T. ) ;
#5946=CARTESIAN_POINT ( 'NONE',  ( 3.756430356250006319, 26.97812499938547859, 6.831223922626973533 ) ) ;
#5949=CARTESIAN_POINT ( 'NONE',  ( 4.000000000000000888, 28.11250000000000426, 11.30940107675849760 ) ) ;
#5950=EDGE_CURVE ( 'NONE', #15046, #13062, #11023, .T. ) ;
#5952=EDGE_CURVE ( 'NONE', #6478, #6543, #7682, .T. ) ;
#5958=EDGE_CURVE ( 'NONE', #930, #17209, #15126, .T. ) ;
#5967=CARTESIAN_POINT ( 'NONE',  ( 6.009258394948636914E-15, 26.26562499938548356, 4.662447845253954171 ) ) ;
#5975=DIRECTION ( 'NONE',  ( 0.000000000000000000, 1.000000000000000000, 0.000000000000000000 ) ) ;
#5976=CARTESIAN_POINT ( 'NONE',  ( 6.009258394948636914E-15, 26.60312499938547859, 4.662447845253954171 ) ) ;
#5981=CARTESIAN_POINT ( 'NONE',  ( 3.469446951953614189E-15, 31.50000000000000000, 8.999999999999992895 ) ) ;
#5984=DIRECTION ( 'NONE',  ( 0.000000000000000000, 0.000000000000000000, -1.000000000000000000 ) ) ;
#5985=CARTESIAN_POINT ( 'NONE',  ( -1.999999999999994893, 26.44374999877097210, 5.535898384862237620 ) ) ;
#5986=DIRECTION ( 'NONE',  ( 0.000000000000000000, 1.000000000000000000, 0.000000000000000000 ) ) ;
#5994=DIRECTION ( 'NONE',  ( -0.000000000000000000, 1.000000000000000000, -0.000000000000000000 ) ) ;
#5997=DIRECTION ( 'NONE',  ( -0.000000000000000000, -1.000000000000000000, -0.000000000000000000 ) ) ;
#6003=ORIENTED_EDGE ( 'NONE', *, *, #9000, .F. ) ;
#6005=EDGE_LOOP ( 'NONE', ( #19144, #3901, #2015, #17719, #4425, #25355, #24586, #6246 ) ) ;
#6009=CARTESIAN_POINT ( 'NONE',  ( -3.023184356956651442, 38.77026726007181878, 13.86739978446106392 ) ) ;
#6011=CARTESIAN_POINT ( 'NONE',  ( 3.756430356250004543, 26.90312499938548996, 11.16877607737301226 ) ) ;
#6012=( GEOMETRIC_REPRESENTATION_CONTEXT ( 3 ) GLOBAL_UNCERTAINTY_ASSIGNED_CONTEXT ( ( #2860 ) ) GLOBAL_UNIT_ASSIGNED_CONTEXT ( ( #7555, #15405, #3626 ) ) REPRESENTATION_CONTEXT ( 'NONE', 'WORKASPACE' ) );
#6026=EDGE_CURVE ( 'NONE', #22395, #12276, #11548, .T. ) ;
#6035=PRODUCT_DEFINITION_FORMATION_WITH_SPECIFIED_SOURCE ( 'ANY', '', #24254, .NOT_KNOWN. ) ;
#6046=CARTESIAN_POINT ( 'NONE',  ( 1.071796769724490783, 25.80759618943233846, 12.99999999999999467 ) ) ;
#6058=CARTESIAN_POINT ( 'NONE',  ( -1.878215178124999829, 26.45312499938549422, 12.25316411605951927 ) ) ;
#6071=CARTESIAN_POINT ( 'NONE',  ( -1.878215178124998275, 29.49062499938548854, 12.25316411605951927 ) ) ;
#6074=CARTESIAN_POINT ( 'NONE',  ( 4.006172263299091013E-15, 29.16250000000000497, 4.381197846482986158 ) ) ;
#6075=LINE ( 'NONE', #14058, #13855 ) ;
#6088=CARTESIAN_POINT ( 'NONE',  ( 1.878215178124999829, 26.97812499938549280, 12.25316411605952283 ) ) ;
#6093=DIRECTION ( 'NONE',  ( 0.000000000000000000, 0.000000000000000000, 1.000000000000000000 ) ) ;
#6096=ORIENTED_EDGE ( 'NONE', *, *, #25170, .T. ) ;
#6098=CARTESIAN_POINT ( 'NONE',  ( 3.756430356250004543, 26.90312499938548996, 11.16877607737301226 ) ) ;
#6104=FACE_OUTER_BOUND ( 'NONE', #13514, .T. ) ;
#6108=CARTESIAN_POINT ( 'NONE',  ( -3.999999999999996447, 26.55624999877097281, 11.30940107675849404 ) ) ;
#6117=CARTESIAN_POINT ( 'NONE',  ( -9.296355089585909904E-15, 29.10624999877097352, 4.999999999999992006 ) ) ;
#6130=CARTESIAN_POINT ( 'NONE',  ( 1.878215178125008489, 26.22812499938548925, 5.746835883940462963 ) ) ;
#6131=( LENGTH_UNIT ( ) NAMED_UNIT ( * ) SI_UNIT ( .MILLI., .METRE. ) );
#6133=CARTESIAN_POINT ( 'NONE',  ( 1.878215178125003382, 26.11562499938548854, 5.746835883940462963 ) ) ;
#6139=LINE ( 'NONE', #13999, #19246 ) ;
#6149=FACE_OUTER_BOUND ( 'NONE', #18414, .T. ) ;
#6161=CARTESIAN_POINT ( 'NONE',  ( 3.469446951953614189E-15, 39.50000000000000000, 8.999999999999992895 ) ) ;
#6165=CARTESIAN_POINT ( 'NONE',  ( 3.469446951953614189E-15, 39.50000000000000000, 8.999999999999992895 ) ) ;
#6167=EDGE_CURVE ( 'NONE', #20633, #6625, #462, .T. ) ;
#6179=CARTESIAN_POINT ( 'NONE',  ( 4.006172263299091013E-15, 25.36562499938549564, 4.662447845253954171 ) ) ;
#6188=EDGE_LOOP ( 'NONE', ( #20771, #24778, #18707, #24693 ) ) ;
#6194=CARTESIAN_POINT ( 'NONE',  ( 0.2821657309629718169, 38.91194779626418665, 3.418731683527081344 ) ) ;
#6195=CARTESIAN_POINT ( 'NONE',  ( 3.469446951953614189E-15, 35.50000000000000711, 8.999999999999992895 ) ) ;
#6213=CARTESIAN_POINT ( 'NONE',  ( -3.756430356249996549, 27.69062499938548072, 6.831223922626973533 ) ) ;
#6216=CARTESIAN_POINT ( 'NONE',  ( 1.071796769724494114, 27.15759618943233988, 12.99999999999999112 ) ) ;
#6218=ORIENTED_EDGE ( 'NONE', *, *, #3370, .T. ) ;
#6221=CARTESIAN_POINT ( 'NONE',  ( -1.878215178124996498, 28.44062499938548783, 5.746835883940462963 ) ) ;
#6246=ORIENTED_EDGE ( 'NONE', *, *, #1611, .F. ) ;
#6252=DIRECTION ( 'NONE',  ( 0.000000000000000000, -0.000000000000000000, 1.000000000000000000 ) ) ;
#6262=CARTESIAN_POINT ( 'NONE',  ( 3.756430356250004543, 25.29062499938548925, 6.831223922626973533 ) ) ;
#6266=CARTESIAN_POINT ( 'NONE',  ( -3.999999999999996447, 28.82500000000000284, 8.999999999999992895 ) ) ;
#6273=CARTESIAN_POINT ( 'NONE',  ( 3.469446951953614189E-15, 35.50000000000000711, 8.999999999999992895 ) ) ;
#6276=CARTESIAN_POINT ( 'NONE',  ( 1.071796769724495446, 26.38615380933864074, 4.999999999999992895 ) ) ;
#6286=ADVANCED_FACE ( 'NONE', ( #22156 ), #4490, .T. ) ;
#6297=AXIS2_PLACEMENT_3D ( 'NONE', #19954, #4281, #2060 ) ;
#6315=EDGE_LOOP ( 'NONE', ( #21342, #20459, #15848, #8384 ) ) ;
#6316=CARTESIAN_POINT ( 'NONE',  ( -3.756430356249996549, 27.27812499938548996, 8.999999999999992895 ) ) ;
#6323=ORIENTED_EDGE ( 'NONE', *, *, #18309, .F. ) ;
#6328=EDGE_LOOP ( 'NONE', ( #11439, #24472, #8731, #17251, #10496, #4062, #7475, #8449, #21067, #17501, #1761, #2449, #1439, #17143, #62, #751 ) ) ;
#6350=CARTESIAN_POINT ( 'NONE',  ( 3.756430356250001434, 27.50312499938548783, 8.999999999999992895 ) ) ;
#6351=ORIENTED_EDGE ( 'NONE', *, *, #9460, .F. ) ;
#6362=CARTESIAN_POINT ( 'NONE',  ( 1.878215178124998275, 26.86562499938548854, 12.25316411605952283 ) ) ;
#6376=ORIENTED_EDGE ( 'NONE', *, *, #17793, .F. ) ;
#6377=CARTESIAN_POINT ( 'NONE',  ( -5.432449689414484695, 38.61000136877622424, 11.27614500780635431 ) ) ;
#6380=AXIS2_PLACEMENT_3D ( 'NONE', #4868, #2776, #816 ) ;
#6396=ORIENTED_EDGE ( 'NONE', *, *, #15366, .T. ) ;
#6397=CARTESIAN_POINT ( 'NONE',  ( -2.003086131649545506E-15, 26.49062499938548143, 13.33755215474602984 ) ) ;
#6423=VERTEX_POINT ( 'NONE', #9453 ) ;
#6427=MECHANICAL_DESIGN_GEOMETRIC_PRESENTATION_REPRESENTATION('',(#16898),#6012);
#6448=CARTESIAN_POINT ( 'NONE',  ( 3.756430356250002323, 28.44062499938549138, 6.831223922626973533 ) ) ;
#6449=EDGE_LOOP ( 'NONE', ( #2809, #5671, #14464, #9784 ) ) ;
#6450=FACE_OUTER_BOUND ( 'NONE', #4028, .T. ) ;
#6452=CARTESIAN_POINT ( 'NONE',  ( 3.469446951953614189E-15, 38.49999999999999289, 8.999999999999992895 ) ) ;
#6454=DIRECTION ( 'NONE',  ( 0.000000000000000000, 1.000000000000000000, 0.000000000000000000 ) ) ;
#6464=CARTESIAN_POINT ( 'NONE',  ( 0.000000000000000000, 28.93750000000000711, 13.61880215351699874 ) ) ;
#6470=CARTESIAN_POINT ( 'NONE',  ( 5.706339097770919189, 29.50000000000000000, 7.145898033750285983 ) ) ;
#6471=FACE_OUTER_BOUND ( 'NONE', #22077, .T. ) ;
#6477=CARTESIAN_POINT ( 'NONE',  ( -3.756430356249994329, 28.59062499938548996, 6.831223922626973533 ) ) ;
#6478=VERTEX_POINT ( 'NONE', #23447 ) ;
#6481=CARTESIAN_POINT ( 'NONE',  ( 3.818666391692735029, 38.64256296259726753, 4.558361811591131740 ) ) ;
#6486=CARTESIAN_POINT ( 'NONE',  ( 1.878215178125001605, 27.31562499938548783, 12.25316411605952283 ) ) ;
#6494=DIRECTION ( 'NONE',  ( -0.000000000000000000, -1.000000000000000000, -0.000000000000000000 ) ) ;
#6511=ORIENTED_EDGE ( 'NONE', *, *, #9258, .T. ) ;
#6513=ORIENTED_EDGE ( 'NONE', *, *, #22970, .F. ) ;
#6529=CARTESIAN_POINT ( 'NONE',  ( 3.469446951953614189E-15, 35.50000000000000711, 8.999999999999992895 ) ) ;
#6533=CARTESIAN_POINT ( 'NONE',  ( -1.999999999999994893, 27.40000000000000213, 5.535898384862237620 ) ) ;
#6543=VERTEX_POINT ( 'NONE', #13902 ) ;
#6548=ORIENTED_EDGE ( 'NONE', *, *, #10109, .T. ) ;
#6569=CARTESIAN_POINT ( 'NONE',  ( -3.756430356249998326, 28.66562499938548925, 11.16877607737301226 ) ) ;
#6584=CARTESIAN_POINT ( 'NONE',  ( -1.999999999999998224, 26.65000000000000568, 12.46410161513774639 ) ) ;
#6591=CARTESIAN_POINT ( 'NONE',  ( -3.999999999999999556, 26.03124999877097423, 6.690598923241487306 ) ) ;
#6599=CARTESIAN_POINT ( 'NONE',  ( 1.878215178125001605, 29.22812499938549280, 12.25316411605952283 ) ) ;
#6606=CARTESIAN_POINT ( 'NONE',  ( -1.878215178124999829, 27.69062499938549138, 12.25316411605951927 ) ) ;
#6609=CARTESIAN_POINT ( 'NONE',  ( -1.878215178124994722, 27.99062499938548143, 5.746835883940462963 ) ) ;
#6610=AXIS2_PLACEMENT_3D ( 'NONE', #14274, #16610, #14517 ) ;
#6625=VERTEX_POINT ( 'NONE', #18298 ) ;
#6632=EDGE_CURVE ( 'NONE', #11238, #19496, #21457, .T. ) ;
#6636=EDGE_CURVE ( 'NONE', #16757, #23529, #17218, .T. ) ;
#6644=CARTESIAN_POINT ( 'NONE',  ( 3.756430356250002323, 26.11562499938549564, 11.16877607737301226 ) ) ;
#6654=AXIS2_PLACEMENT_3D ( 'NONE', #8607, #18558, #2597 ) ;
#6668=ORIENTED_EDGE ( 'NONE', *, *, #5952, .F. ) ;
#6694=CARTESIAN_POINT ( 'NONE',  ( 2.000000000000005329, 25.46874999877096712, 5.535898384862238508 ) ) ;
#6698=CARTESIAN_POINT ( 'NONE',  ( 3.756430356250004543, 28.89062499938549067, 6.831223922626973533 ) ) ;
#6705=LINE ( 'NONE', #16652, #2162 ) ;
#6726=CARTESIAN_POINT ( 'NONE',  ( 4.000000000000000888, 26.25624999877096144, 11.30940107675849760 ) ) ;
#6730=CARTESIAN_POINT ( 'NONE',  ( 5.840899737312979845, 38.49999999999999289, 10.37254881831474052 ) ) ;
#6735=CARTESIAN_POINT ( 'NONE',  ( 3.756430356250000546, 29.26562499938548356, 11.16877607737301403 ) ) ;
#6741=DIRECTION ( 'NONE',  ( -0.000000000000000000, -1.000000000000000000, -0.000000000000000000 ) ) ;
#6745=CARTESIAN_POINT ( 'NONE',  ( -3.756430356249996549, 25.32812499938548356, 6.831223922626973533 ) ) ;
#6749=CARTESIAN_POINT ( 'NONE',  ( 3.756430356250004543, 26.07812499938549422, 6.831223922626973533 ) ) ;
#6771=CARTESIAN_POINT ( 'NONE',  ( 3.756430356250004987, 29.69687499938549280, 8.999999999999992895 ) ) ;
#6782=ORIENTED_EDGE ( 'NONE', *, *, #22216, .F. ) ;
#6785=CARTESIAN_POINT ( 'NONE',  ( 3.756430356250002323, 27.46562499938548640, 11.16877607737301226 ) ) ;
#6789=EDGE_CURVE ( 'NONE', #25495, #10104, #24297, .T. ) ;
#6790=CARTESIAN_POINT ( 'NONE',  ( -3.202926563175272801, 39.00162299460587434, 4.530527552673861535 ) ) ;
#6795=CARTESIAN_POINT ( 'NONE',  ( 3.110308778861350820, 31.50000000000000000, 14.13088484572962855 ) ) ;
#6819=CARTESIAN_POINT ( 'NONE',  ( 4.000000000000001776, 29.50000000000000711, 8.999999999999992895 ) ) ;
#6825=DIRECTION ( 'NONE',  ( -0.000000000000000000, -1.000000000000000000, -0.000000000000000000 ) ) ;
#6828=DIRECTION ( 'NONE',  ( -0.000000000000000000, 1.000000000000000000, -0.000000000000000000 ) ) ;
#6830=CARTESIAN_POINT ( 'NONE',  ( 1.533898589781675205E-14, 27.98124999877097352, 12.99999999999999289 ) ) ;
#6832=CARTESIAN_POINT ( 'NONE',  ( -3.999999999999998224, 28.76874999877097139, 8.999999999999992895 ) ) ;
#6836=CARTESIAN_POINT ( 'NONE',  ( 3.469446951953614189E-15, 35.50000000000000711, 4.999999999999992006 ) ) ;
#6839=CARTESIAN_POINT ( 'NONE',  ( 3.756430356250006319, 27.09062499938548285, 6.831223922626973533 ) ) ;
#6855=EDGE_CURVE ( 'NONE', #4270, #6478, #6705, .T. ) ;
#6858=EDGE_CURVE ( 'NONE', #6625, #13467, #7092, .T. ) ;
#6863=CARTESIAN_POINT ( 'NONE',  ( -3.999999999999996447, 26.55624999877097281, 11.30940107675849404 ) ) ;
#6869=CARTESIAN_POINT ( 'NONE',  ( 3.756430356250003211, 28.85312499938548569, 8.999999999999992895 ) ) ;
#6877=CARTESIAN_POINT ( 'NONE',  ( -1.878215178124998275, 26.79062499938548569, 12.25316411605951927 ) ) ;
#6879=CARTESIAN_POINT ( 'NONE',  ( -3.756430356249996105, 28.47812499938548569, 6.831223922626973533 ) ) ;
#6896=ORIENTED_EDGE ( 'NONE', *, *, #1789, .T. ) ;
#6909=CARTESIAN_POINT ( 'NONE',  ( -3.756430356249994329, 26.79062499938549280, 6.831223922626973533 ) ) ;
#6914=CARTESIAN_POINT ( 'NONE',  ( -3.434389267989125027, 38.94985767598075910, 4.639816847356652119 ) ) ;
#6936=( BOUNDED_CURVE ( )  B_SPLINE_CURVE ( 2, ( #23137, #21049, #9653, #21428, #1676, #17121, #1290, #3375, #19071 ),
 .UNSPECIFIED., .F., .F. ) 
 B_SPLINE_CURVE_WITH_KNOTS ( ( 3, 2, 2, 2, 3 ),
 ( 0.8750000000000000000, 0.8833333333333333037, 0.9000000000000000222, 0.9166666666666666297, 0.9250000000000000444 ),
 .UNSPECIFIED. ) 
 CURVE ( )  GEOMETRIC_REPRESENTATION_ITEM ( )  RATIONAL_B_SPLINE_CURVE ( ( 0.9330127018922194093, 0.9330127018922194093, 1.000000000000000000, 0.8660254037844387076, 1.000000000000000000, 0.8660254037844387076, 1.000000000000000000, 0.9330127018922189652, 0.9330127018922194093 ) ) 
 REPRESENTATION_ITEM ( '' )  );
#6943=( BOUNDED_CURVE ( )  B_SPLINE_CURVE ( 2, ( #19813, #25581, #5695, #13674, #3728, #11712, #19689, #7787, #9248 ),
 .UNSPECIFIED., .F., .T. ) 
 B_SPLINE_CURVE_WITH_KNOTS ( ( 3, 2, 2, 2, 3 ),
 ( 0.3750000000000000000, 0.3833333333333333592, 0.4000000000000000222, 0.4166666666666666852, 0.4250000000000000444 ),
 .UNSPECIFIED. ) 
 CURVE ( )  GEOMETRIC_REPRESENTATION_ITEM ( )  RATIONAL_B_SPLINE_CURVE ( ( 0.9330127018922194093, 0.9330127018922194093, 1.000000000000000000, 0.8660254037844387076, 1.000000000000000000, 0.8660254037844387076, 1.000000000000000000, 0.9330127018922191873, 0.9330127018922194093 ) ) 
 REPRESENTATION_ITEM ( '' )  );
#6984=CARTESIAN_POINT ( 'NONE',  ( 4.000000000000005329, 28.09374999877097778, 8.999999999999992895 ) ) ;
#6989=CARTESIAN_POINT ( 'NONE',  ( -1.878215178124996498, 29.00312499938548783, 5.746835883940462963 ) ) ;
#6999=CARTESIAN_POINT ( 'NONE',  ( -3.756430356250000546, 26.30312499938548854, 11.16877607737301048 ) ) ;
#7001=CARTESIAN_POINT ( 'NONE',  ( 3.756430356250002323, 28.32812499938549067, 6.831223922626973533 ) ) ;
#7003=CARTESIAN_POINT ( 'NONE',  ( 5.706339097770919189, 31.50000000000000000, 7.145898033750285983 ) ) ;
#7017=AXIS2_PLACEMENT_3D ( 'NONE', #22355, #20525, #4439 ) ;
#7030=CARTESIAN_POINT ( 'NONE',  ( 6.009258394948636914E-15, 27.61562499938548854, 4.662447845253954171 ) ) ;
#7032=ADVANCED_FACE ( 'NONE', ( #1351 ), #19633, .T. ) ;
#7038=CARTESIAN_POINT ( 'NONE',  ( -3.338796519864625445, 38.98631256281465340, 4.611909993434559318 ) ) ;
#7057=CARTESIAN_POINT ( 'NONE',  ( -5.500712606062064580, 38.82887297708774810, 7.617000894021300539 ) ) ;
#7062=ORIENTED_EDGE ( 'NONE', *, *, #17841, .F. ) ;
#7063=ORIENTED_EDGE ( 'NONE', *, *, #10001, .F. ) ;
#7064=ORIENTED_EDGE ( 'NONE', *, *, #15329, .F. ) ;
#7065=LINE ( 'NONE', #23158, #11791 ) ;
#7080=CARTESIAN_POINT ( 'NONE',  ( 3.918623196469491976, 38.49999999999999289, 13.54361004533742907 ) ) ;
#7083=DIRECTION ( 'NONE',  ( -0.000000000000000000, 1.000000000000000000, -0.000000000000000000 ) ) ;
#7092=( BOUNDED_CURVE ( )  B_SPLINE_CURVE ( 2, ( #2917, #704, #8805, #20577, #10497, #25011, #16924, #9059, #10749 ),
 .UNSPECIFIED., .F., .F. ) 
 B_SPLINE_CURVE_WITH_KNOTS ( ( 3, 2, 2, 2, 3 ),
 ( 0.5250000000000000222, 0.5333333333333333259, 0.5500000000000000444, 0.5666666666666666519, 0.5750000000000000666 ),
 .UNSPECIFIED. ) 
 CURVE ( )  GEOMETRIC_REPRESENTATION_ITEM ( )  RATIONAL_B_SPLINE_CURVE ( ( 0.9330127018922194093, 0.9330127018922194093, 1.000000000000000000, 0.8660254037844387076, 1.000000000000000000, 0.8660254037844387076, 1.000000000000000000, 0.9330127018922189652, 0.9330127018922194093 ) ) 
 REPRESENTATION_ITEM ( '' )  );
#7116=AXIS2_PLACEMENT_3D ( 'NONE', #21013, #25194, #21130 ) ;
#7121=CARTESIAN_POINT ( 'NONE',  ( 2.000000000000003553, 27.71874999877097778, 5.535898384862238508 ) ) ;
#7127=CARTESIAN_POINT ( 'NONE',  ( -3.756430356249997882, 29.04062499938548569, 6.831223922626973533 ) ) ;
#7129=ORIENTED_EDGE ( 'NONE', *, *, #2128, .T. ) ;
#7137=CARTESIAN_POINT ( 'NONE',  ( -3.756430356249994773, 25.81562499938548783, 8.999999999999992895 ) ) ;
#7140=CARTESIAN_POINT ( 'NONE',  ( 1.878215178125001605, 28.66562499938549280, 12.25316411605952283 ) ) ;
#7164=ADVANCED_FACE ( 'NONE', ( #20951 ), #24871, .F. ) ;
#7173=CARTESIAN_POINT ( 'NONE',  ( 3.756430356250002323, 28.44062499938549138, 6.831223922626973533 ) ) ;
#7179=CARTESIAN_POINT ( 'NONE',  ( 4.000000000000002665, 28.56249999999999645, 11.30940107675849760 ) ) ;
#7223=ADVANCED_FACE ( 'NONE', ( #15894 ), #3717, .T. ) ;
#7230=ORIENTED_EDGE ( 'NONE', *, *, #22294, .T. ) ;
#7234=EDGE_CURVE ( 'NONE', #10411, #25139, #6075, .T. ) ;
#7243=CARTESIAN_POINT ( 'NONE',  ( 4.648177544792955347E-16, 25.78750000000000497, 12.99999999999999289 ) ) ;
#7253=CARTESIAN_POINT ( 'NONE',  ( -1.999999999999994893, 27.79374999877096997, 5.535898384862237620 ) ) ;
#7256=MECHANICAL_DESIGN_GEOMETRIC_PRESENTATION_REPRESENTATION('',(#587),#17700);
#7260=DIRECTION ( 'NONE',  ( 0.000000000000000000, -0.7071067811865503483, -0.7071067811865446862 ) ) ;
#7274=CARTESIAN_POINT ( 'NONE',  ( -3.756430356250000546, 28.55312499938549564, 11.16877607737301226 ) ) ;
#7280=CARTESIAN_POINT ( 'NONE',  ( -3.999999999999996447, 27.00624999877097565, 11.30940107675849404 ) ) ;
#7296=VERTEX_POINT ( 'NONE', #14543 ) ;
#7301=CARTESIAN_POINT ( 'NONE',  ( -1.878215178124999829, 28.70312499938548711, 12.25316411605951927 ) ) ;
#7315=DIRECTION ( 'NONE',  ( -0.000000000000000000, -1.000000000000000000, -0.000000000000000000 ) ) ;
#7320=CARTESIAN_POINT ( 'NONE',  ( 3.469446951953614189E-15, 38.49999999999999289, 8.999999999999992895 ) ) ;
#7325=ORIENTED_EDGE ( 'NONE', *, *, #14470, .F. ) ;
#7330=CARTESIAN_POINT ( 'NONE',  ( 4.006172263299091013E-15, 25.25312499938549138, 4.662447845253954171 ) ) ;
#7338=LINE ( 'NONE', #15447, #10511 ) ;
#7343=CARTESIAN_POINT ( 'NONE',  ( 3.959305671612554781E-15, 35.50000000000000711, 12.99999999999999289 ) ) ;
#7358=ORIENTED_EDGE ( 'NONE', *, *, #2378, .T. ) ;
#7373=CARTESIAN_POINT ( 'NONE',  ( 4.000000000000003553, 28.54374999877097707, 8.999999999999992895 ) ) ;
#7387=CARTESIAN_POINT ( 'NONE',  ( 8.012344526598182026E-15, 27.05312499938548854, 4.662447845253954171 ) ) ;
#7389=CARTESIAN_POINT ( 'NONE',  ( -1.878215178124996498, 28.44062499938548783, 5.746835883940462963 ) ) ;
#7399=EDGE_CURVE ( 'NONE', #32, #16533, #11745, .T. ) ;
#7409=CARTESIAN_POINT ( 'NONE',  ( -2.003086131649545506E-15, 26.04062499938549280, 13.33755215474603162 ) ) ;
#7410=VERTEX_POINT ( 'NONE', #16637 ) ;
#7412=VERTEX_POINT ( 'NONE', #16522 ) ;
#7415=ORIENTED_EDGE ( 'NONE', *, *, #2634, .T. ) ;
#7417=CARTESIAN_POINT ( 'NONE',  ( 3.756430356250003211, 25.59062499938548285, 8.999999999999992895 ) ) ;
#7422=CARTESIAN_POINT ( 'NONE',  ( 1.071796769724495002, 26.89240381056767504, 4.999999999999989342 ) ) ;
#7475=ORIENTED_EDGE ( 'NONE', *, *, #19884, .F. ) ;
#7493=DIRECTION ( 'NONE',  ( 8.659560562354900811E-17, -0.7071067811865503483, 0.7071067811865446862 ) ) ;
#7497=CARTESIAN_POINT ( 'NONE',  ( -3.999999999999999556, 27.90624999877097778, 11.30940107675849404 ) ) ;
#7503=ADVANCED_FACE ( 'NONE', ( #17296 ), #16912, .F. ) ;
#7506=VERTEX_POINT ( 'NONE', #12973 ) ;
#7513=CARTESIAN_POINT ( 'NONE',  ( 3.756430356250002323, 28.32812499938548356, 6.831223922626973533 ) ) ;
#7515=CARTESIAN_POINT ( 'NONE',  ( 3.469446951953614189E-15, 35.50000000000000711, 4.999999999999992006 ) ) ;
#7516=CARTESIAN_POINT ( 'NONE',  ( 4.000000000000005329, 26.80000000000000426, 8.999999999999992895 ) ) ;
#7522=CARTESIAN_POINT ( 'NONE',  ( 3.878215178125003604, 29.82343749907823138, 8.999999999999992895 ) ) ;
#7524=EDGE_CURVE ( 'NONE', #11405, #22637, #4247, .T. ) ;
#7529=AXIS2_PLACEMENT_3D ( 'NONE', #23356, #17863, #5580 ) ;
#7530=EDGE_CURVE ( 'NONE', #15689, #22370, #23361, .T. ) ;
#7532=CARTESIAN_POINT ( 'NONE',  ( 4.000000000000001776, 25.84374999877097423, 8.999999999999992895 ) ) ;
#7547=CARTESIAN_POINT ( 'NONE',  ( 3.756430356250003211, 26.04062499938548925, 8.999999999999992895 ) ) ;
#7555=( LENGTH_UNIT ( ) NAMED_UNIT ( * ) SI_UNIT ( .MILLI., .METRE. ) );
#7559=CARTESIAN_POINT ( 'NONE',  ( 1.071796769724490783, 28.50759618943234130, 12.99999999999999467 ) ) ;
#7574=CARTESIAN_POINT ( 'NONE',  ( -1.878215178124998275, 29.60312499938548925, 12.25316411605951927 ) ) ;
#7577=ORIENTED_EDGE ( 'NONE', *, *, #12078, .T. ) ;
#7578=CIRCLE ( 'NONE', #20088, 4.000000000000000000 ) ;
#7590=EDGE_CURVE ( 'NONE', #13124, #486, #9311, .T. ) ;
#7598=CARTESIAN_POINT ( 'NONE',  ( 0.4995657836784154204, 38.49999999999999289, 3.020833333333325044 ) ) ;
#7602=CARTESIAN_POINT ( 'NONE',  ( 1.071796769724498111, 27.60759618943233207, 12.99999999999998757 ) ) ;
#7609=DIRECTION ( 'NONE',  ( 0.000000000000000000, -1.000000000000000000, 0.000000000000000000 ) ) ;
#7610=ORIENTED_EDGE ( 'NONE', *, *, #22730, .T. ) ;
#7634=CARTESIAN_POINT ( 'NONE',  ( 2.000000000000000000, 28.07500000000000995, 12.46410161513774817 ) ) ;
#7637=CARTESIAN_POINT ( 'NONE',  ( 1.878215178125003382, 25.32812499938548356, 5.746835883940462963 ) ) ;
#7643=ORIENTED_EDGE ( 'NONE', *, *, #15801, .T. ) ;
#7647=CARTESIAN_POINT ( 'NONE',  ( -1.998723687422152831E-12, 39.00000000001113420, 14.49999999998978240 ) ) ;
#7648=EDGE_CURVE ( 'NONE', #13124, #20633, #12431, .T. ) ;
#7650=CARTESIAN_POINT ( 'NONE',  ( -1.878215178124998275, 28.14062499938548711, 12.25316411605951927 ) ) ;
#7652=CARTESIAN_POINT ( 'NONE',  ( 4.000000000000002665, 27.66249999999999787, 11.30940107675849760 ) ) ;
#7657=EDGE_CURVE ( 'NONE', #11405, #11752, #13472, .T. ) ;
#7672=CARTESIAN_POINT ( 'NONE',  ( -3.756430356249997882, 25.51562499938549067, 11.16877607737301048 ) ) ;
#7680=ORIENTED_EDGE ( 'NONE', *, *, #22902, .F. ) ;
#7681=CARTESIAN_POINT ( 'NONE',  ( -3.756430356249997882, 26.26562499938548711, 8.999999999999992895 ) ) ;
#7682=CIRCLE ( 'NONE', #22607, 4.000000000000000000 ) ;
#7686=CARTESIAN_POINT ( 'NONE',  ( 0.4995657836784084815, 34.50000000000000000, 14.97916666666665897 ) ) ;
#7688=CARTESIAN_POINT ( 'NONE',  ( 2.000000000000000000, 28.52500000000000924, 12.46410161513774817 ) ) ;
#7701=DIRECTION ( 'NONE',  ( -0.000000000000000000, -1.000000000000000000, -0.000000000000000000 ) ) ;
#7717=CARTESIAN_POINT ( 'NONE',  ( -3.756430356249996105, 25.40312499938548640, 11.16877607737301226 ) ) ;
#7726=CARTESIAN_POINT ( 'NONE',  ( 2.000000000000005329, 27.77500000000000568, 5.535898384862238508 ) ) ;
#7730=LINE ( 'NONE', #19761, #22474 ) ;
#7746=CARTESIAN_POINT ( 'NONE',  ( 2.000000000000000000, 29.42500000000000426, 12.46410161513774817 ) ) ;
#7750=VECTOR ( 'NONE', #558, 1000.000000000000000 ) ;
#7761=CARTESIAN_POINT ( 'NONE',  ( -1.878215178124998275, 26.00312499938549493, 12.25316411605951927 ) ) ;
#7773=CARTESIAN_POINT ( 'NONE',  ( 3.202063662808456446, 39.00157412423376968, 4.529845232042116976 ) ) ;
#7775=( BOUNDED_CURVE ( )  B_SPLINE_CURVE ( 2, ( #10113, #18114, #17714, #189, #21620, #3703, #11684, #23709, #5795 ),
 .UNSPECIFIED., .F., .F. ) 
 B_SPLINE_CURVE_WITH_KNOTS ( ( 3, 2, 2, 2, 3 ),
 ( 0.9250000000000000444, 0.9333333333333333481, 0.9499999999999999556, 0.9666666666666666741, 0.9749999999999999778 ),
 .UNSPECIFIED. ) 
 CURVE ( )  GEOMETRIC_REPRESENTATION_ITEM ( )  RATIONAL_B_SPLINE_CURVE ( ( 0.9330127018922194093, 0.9330127018922198534, 1.000000000000000000, 0.8660254037844387076, 1.000000000000000000, 0.8660254037844387076, 1.000000000000000000, 0.9330127018922194093, 0.9330127018922194093 ) ) 
 REPRESENTATION_ITEM ( '' )  );
#7776=CARTESIAN_POINT ( 'NONE',  ( -3.756430356250000546, 28.55312499938548854, 11.16877607737301048 ) ) ;
#7778=CARTESIAN_POINT ( 'NONE',  ( -1.999999999999998224, 26.95000000000000639, 5.535898384862237620 ) ) ;
#7787=CARTESIAN_POINT ( 'NONE',  ( 1.071796769724492115, 27.28615380933864287, 4.999999999999989342 ) ) ;
#7788=ADVANCED_FACE ( 'NONE', ( #14398 ), #20660, .F. ) ;
#7803=CARTESIAN_POINT ( 'NONE',  ( -3.756430356249996105, 25.32812499938549067, 6.831223922626973533 ) ) ;
#7806=B_SPLINE_CURVE_WITH_KNOTS ( 'NONE', 3,
 ( #10630, #18621, #22406, #24106, #2282, #8675, #14180, #22150 ),
 .UNSPECIFIED., .F., .F.,
 ( 4, 2, 2, 4 ),
 ( 0.0009289288217882851880, 0.001160777380751508870, 0.001392625939714732444, 0.001856323057641176772 ),
 .UNSPECIFIED. ) ;
#7811=CARTESIAN_POINT ( 'NONE',  ( 4.648177544792955347E-16, 29.33124999877097139, 12.99999999999999289 ) ) ;
#7813=CYLINDRICAL_SURFACE ( 'NONE', #20830, 0.5000000000000004441 ) ;
#7817=CARTESIAN_POINT ( 'NONE',  ( -5.206645097256043186, 38.99989214654020486, 10.77428791256852669 ) ) ;
#7833=CARTESIAN_POINT ( 'NONE',  ( -9.296355089585910693E-16, 26.91250000000000497, 4.999999999999991118 ) ) ;
#7836=CARTESIAN_POINT ( 'NONE',  ( -1.878215178124996498, 27.54062499938548569, 5.746835883940462963 ) ) ;
#7842=DIRECTION ( 'NONE',  ( 0.000000000000000000, 0.000000000000000000, -1.000000000000000000 ) ) ;
#7845=CARTESIAN_POINT ( 'NONE',  ( 5.112995299272250684E-15, 26.40624999877096712, 4.999999999999992006 ) ) ;
#7875=CARTESIAN_POINT ( 'NONE',  ( 5.577813053751546416E-15, 25.33750000000000924, 12.99999999999999289 ) ) ;
#7883=CARTESIAN_POINT ( 'NONE',  ( 3.756430356250004987, 25.25312499938548427, 8.999999999999992895 ) ) ;
#7896=CARTESIAN_POINT ( 'NONE',  ( 3.027510705461079255, 38.86058378564762705, 4.241563202499551544 ) ) ;
#7898=CARTESIAN_POINT ( 'NONE',  ( 3.756430356250004099, 29.22812499938548569, 6.831223922626973533 ) ) ;
#7901=CARTESIAN_POINT ( 'NONE',  ( 4.000000000000005329, 26.83750000000000213, 6.690598923241489970 ) ) ;
#7922=CARTESIAN_POINT ( 'NONE',  ( 3.756430356250004099, 26.19062499938549138, 6.831223922626973533 ) ) ;
#7932=DIRECTION ( 'NONE',  ( 0.000000000000000000, 0.000000000000000000, 1.000000000000000000 ) ) ;
#7933=CARTESIAN_POINT ( 'NONE',  ( 1.878215178125006934, 26.56562499938548783, 5.746835883940462963 ) ) ;
#7940=CYLINDRICAL_SURFACE ( 'NONE', #8876, 6.000000000000000888 ) ;
#7950=FACE_OUTER_BOUND ( 'NONE', #10739, .T. ) ;
#7951=CARTESIAN_POINT ( 'NONE',  ( 5.532151103383234236, 38.49999999999999289, 6.677220593914319657 ) ) ;
#7956=CARTESIAN_POINT ( 'NONE',  ( -3.999999999999998224, 26.12500000000001066, 8.999999999999992895 ) ) ;
#7975=CARTESIAN_POINT ( 'NONE',  ( -3.756430356250000546, 26.75312499938548783, 11.16877607737301226 ) ) ;
#8002=ORIENTED_EDGE ( 'NONE', *, *, #5950, .T. ) ;
#8011=AXIS2_PLACEMENT_3D ( 'NONE', #18988, #7083, #1073 ) ;
#8019=CYLINDRICAL_SURFACE ( 'NONE', #15896, 6.000000000000000888 ) ;
#8022=CARTESIAN_POINT ( 'NONE',  ( 5.706339097770919189, 31.50000000000000000, 7.145898033750285983 ) ) ;
#8024=ORIENTED_EDGE ( 'NONE', *, *, #14498, .F. ) ;
#8026=CARTESIAN_POINT ( 'NONE',  ( 2.000000000000003553, 29.06874999877097210, 5.535898384862238508 ) ) ;
#8038=CARTESIAN_POINT ( 'NONE',  ( -1.999999999999993117, 25.99374999877097281, 5.535898384862237620 ) ) ;
#8047=CARTESIAN_POINT ( 'NONE',  ( -3.999999999999999556, 27.51250000000000639, 11.30940107675849404 ) ) ;
#8064=CARTESIAN_POINT ( 'NONE',  ( 3.756430356250000546, 26.56562499938549138, 11.16877607737301403 ) ) ;
#8074=CARTESIAN_POINT ( 'NONE',  ( 6.009258394948636914E-15, 27.95312499938548356, 4.662447845253954171 ) ) ;
#8079=( BOUNDED_CURVE ( )  B_SPLINE_CURVE ( 2, ( #3628, #7559, #7688, #7179, #11480, #5216, #15671, #13579, #13072 ),
 .UNSPECIFIED., .F., .F. ) 
 B_SPLINE_CURVE_WITH_KNOTS ( ( 3, 2, 2, 2, 3 ),
 ( 0.7750000000000000222, 0.7833333333333333259, 0.8000000000000000444, 0.8166666666666666519, 0.8250000000000000666 ),
 .UNSPECIFIED. ) 
 CURVE ( )  GEOMETRIC_REPRESENTATION_ITEM ( )  RATIONAL_B_SPLINE_CURVE ( ( 0.9330127018922194093, 0.9330127018922194093, 1.000000000000000000, 0.8660254037844387076, 1.000000000000000000, 0.8660254037844387076, 1.000000000000000000, 0.9330127018922189652, 0.9330127018922194093 ) ) 
 REPRESENTATION_ITEM ( '' )  );
#8081=CARTESIAN_POINT ( 'NONE',  ( -5.706339097770935176, 31.50000000000000000, 7.645898033750358813 ) ) ;
#8089=CARTESIAN_POINT ( 'NONE',  ( 5.326315416280042569, 38.74360394679613506, 6.816580744743770737 ) ) ;
#8094=CARTESIAN_POINT ( 'NONE',  ( 7.901901826148023498E-15, 26.23750000000000426, 12.99999999999999112 ) ) ;
#8105=EDGE_LOOP ( 'NONE', ( #9943, #19178, #22501, #11916 ) ) ;
#8112=CARTESIAN_POINT ( 'NONE',  ( -3.756430356249997882, 26.26562499938548711, 8.999999999999992895 ) ) ;
#8125=CARTESIAN_POINT ( 'NONE',  ( 5.577813053751546416E-15, 28.20624999877096784, 4.999999999999992006 ) ) ;
#8133=VERTEX_POINT ( 'NONE', #11740 ) ;
#8138=ORIENTED_EDGE ( 'NONE', *, *, #3482, .T. ) ;
#8152=CARTESIAN_POINT ( 'NONE',  ( 4.648177544792954952E-15, 28.26250000000000284, 4.999999999999992006 ) ) ;
#8155=CARTESIAN_POINT ( 'NONE',  ( -1.999999999999996669, 29.74374999877097636, 12.46410161513774639 ) ) ;
#8169=CARTESIAN_POINT ( 'NONE',  ( -3.756430356249996549, 29.37812499938548427, 6.831223922626973533 ) ) ;
#8171=CARTESIAN_POINT ( 'NONE',  ( -1.071796769724489451, 26.48259618943233562, 4.999999999999992895 ) ) ;
#8172=CARTESIAN_POINT ( 'NONE',  ( 2.000000000000005329, 28.67500000000000426, 5.535898384862238508 ) ) ;
#8176=DIRECTION ( 'NONE',  ( 0.000000000000000000, 1.000000000000000000, -0.000000000000000000 ) ) ;
#8183=ORIENTED_EDGE ( 'NONE', *, *, #14768, .T. ) ;
#8186=CARTESIAN_POINT ( 'NONE',  ( -1.878215178124996498, 27.20312499938549067, 5.746835883940462963 ) ) ;
#8187=ORIENTED_EDGE ( 'NONE', *, *, #23256, .F. ) ;
#8195=CARTESIAN_POINT ( 'NONE',  ( 3.756430356250002323, 28.25312499938548783, 11.16877607737301226 ) ) ;
#8197=ADVANCED_FACE ( 'NONE', ( #21909 ), #10131, .F. ) ;
#8200=CARTESIAN_POINT ( 'NONE',  ( -3.999999999999998224, 28.31874999877097210, 8.999999999999992895 ) ) ;
#8216=CARTESIAN_POINT ( 'NONE',  ( -1.071796769724488785, 29.31115380933864145, 12.99999999999999289 ) ) ;
#8220=FACE_OUTER_BOUND ( 'NONE', #20418, .T. ) ;
#8230=CARTESIAN_POINT ( 'NONE',  ( -3.756430356249994773, 28.06562499938548783, 8.999999999999992895 ) ) ;
#8231=CARTESIAN_POINT ( 'NONE',  ( -7.901901826148023498E-15, 28.71250000000000568, 4.999999999999992006 ) ) ;
#8234=( BOUNDED_CURVE ( )  B_SPLINE_CURVE ( 2, ( #7811, #15931, #21813, #23903, #20096, #19955, #15672, #5851, #3896 ),
 .UNSPECIFIED., .F., .T. ) 
 B_SPLINE_CURVE_WITH_KNOTS ( ( 3, 2, 2, 2, 3 ),
 ( 0.8750000000000000000, 0.8833333333333333037, 0.9000000000000000222, 0.9166666666666666297, 0.9250000000000000444 ),
 .UNSPECIFIED. ) 
 CURVE ( )  GEOMETRIC_REPRESENTATION_ITEM ( )  RATIONAL_B_SPLINE_CURVE ( ( 0.9330127018922194093, 0.9330127018922194093, 1.000000000000000000, 0.8660254037844387076, 1.000000000000000000, 0.8660254037844387076, 1.000000000000000000, 0.9330127018922189652, 0.9330127018922194093 ) ) 
 REPRESENTATION_ITEM ( '' )  );
#8253=ORIENTED_EDGE ( 'NONE', *, *, #12763, .T. ) ;
#8255=ORIENTED_EDGE ( 'NONE', *, *, #10394, .F. ) ;
#8259=VERTEX_POINT ( 'NONE', #2030 ) ;
#8266=EDGE_CURVE ( 'NONE', #11238, #32, #14064, .T. ) ;
#8278=CARTESIAN_POINT ( 'NONE',  ( -3.756430356249998326, 27.24062499938548854, 6.831223922626973533 ) ) ;
#8290=DIRECTION ( 'NONE',  ( 0.8660254037844395958, -0.4999999999999982236, 0.000000000000000000 ) ) ;
#8294=CARTESIAN_POINT ( 'NONE',  ( -1.999999999999998224, 28.30000000000000426, 5.535898384862237620 ) ) ;
#8302=DIRECTION ( 'NONE',  ( 0.000000000000000000, 1.000000000000000000, 0.000000000000000000 ) ) ;
#8310=CARTESIAN_POINT ( 'NONE',  ( 1.878215178125003382, 28.02812499938548996, 5.746835883940462963 ) ) ;
#8318=CARTESIAN_POINT ( 'NONE',  ( 1.878215178125001605, 28.66562499938549280, 12.25316411605952283 ) ) ;
#8329=AXIS2_PLACEMENT_3D ( 'NONE', #8685, #7609, #3551 ) ;
#8356=CARTESIAN_POINT ( 'NONE',  ( 2.003086131649545506E-15, 25.59062499938548996, 13.33755215474602984 ) ) ;
#8360=CARTESIAN_POINT ( 'NONE',  ( -1.071796769724489895, 28.91740381056767362, 12.99999999999999289 ) ) ;
#8374=VECTOR ( 'NONE', #24617, 1000.000000000000000 ) ;
#8384=ORIENTED_EDGE ( 'NONE', *, *, #6167, .F. ) ;
#8414=CARTESIAN_POINT ( 'NONE',  ( -3.756430356249994329, 26.86562499938548498, 11.16877607737301226 ) ) ;
#8433=CARTESIAN_POINT ( 'NONE',  ( 2.000000000000000000, 28.97500000000000853, 12.46410161513774817 ) ) ;
#8438=DIRECTION ( 'NONE',  ( 0.000000000000000000, 1.000000000000000000, 0.000000000000000000 ) ) ;
#8443=LINE ( 'NONE', #87, #9571 ) ;
#8444=CARTESIAN_POINT ( 'NONE',  ( 5.220798168720365062, 38.91217497027906802, 10.99271487579059325 ) ) ;
#8448=CARTESIAN_POINT ( 'NONE',  ( 3.756430356250002323, 27.91562499938548925, 11.16877607737301403 ) ) ;
#8449=ORIENTED_EDGE ( 'NONE', *, *, #15924, .F. ) ;
#8454=CARTESIAN_POINT ( 'NONE',  ( 3.874318223440419207, 38.57128445889050283, 4.512312944482766319 ) ) ;
#8459=CARTESIAN_POINT ( 'NONE',  ( -3.756430356250000546, 28.55312499938549564, 11.16877607737301226 ) ) ;
#8464=FACE_OUTER_BOUND ( 'NONE', #2047, .T. ) ;
#8493=CARTESIAN_POINT ( 'NONE',  ( 3.110308778861349932, 38.49999999999999289, 14.13088484572963033 ) ) ;
#8504=LINE ( 'NONE', #16486, #15508 ) ;
#8510=ADVANCED_FACE ( 'NONE', ( #15592 ), #11907, .T. ) ;
#8518=CYLINDRICAL_SURFACE ( 'NONE', #1240, 6.000000000000000888 ) ;
#8526=ORIENTED_EDGE ( 'NONE', *, *, #604, .F. ) ;
#8541=CARTESIAN_POINT ( 'NONE',  ( -3.999999999999996447, 28.80624999877097281, 11.30940107675849404 ) ) ;
#8547=CARTESIAN_POINT ( 'NONE',  ( 3.756430356250003211, 28.40312499938548640, 8.999999999999992895 ) ) ;
#8549=CARTESIAN_POINT ( 'NONE',  ( 3.469446951953614189E-15, 35.50000000000000711, 8.999999999999992895 ) ) ;
#8551=B_SPLINE_CURVE_WITH_KNOTS ( 'NONE', 3,
 ( #2997, #530, #6914, #7038, #18819, #6790, #18951, #1036, #18571, #9010, #24837, #12682, #14640, #10696 ),
 .UNSPECIFIED., .F., .F.,
 ( 4, 2, 2, 2, 2, 2, 4 ),
 ( 0.0005975277179059593300, 0.0007548771353729052036, 0.0009122265528398510771, 0.001069575970306796842, 0.001226925387773742824, 0.001541624222707645197, 0.001856323057641547569 ),
 .UNSPECIFIED. ) ;
#8553=ORIENTED_EDGE ( 'NONE', *, *, #19593, .T. ) ;
#8558=CARTESIAN_POINT ( 'NONE',  ( 6.009258394948636914E-15, 29.30312499938549564, 4.662447845253954171 ) ) ;
#8564=ADVANCED_FACE ( 'NONE', ( #6149 ), #13883, .F. ) ;
#8569=CARTESIAN_POINT ( 'NONE',  ( 5.706339097770929847, 31.50000000000000000, 10.85410196624966517 ) ) ;
#8573=ORIENTED_EDGE ( 'NONE', *, *, #5167, .T. ) ;
#8576=CARTESIAN_POINT ( 'NONE',  ( 3.756430356250004099, 27.54062499938548569, 6.831223922626973533 ) ) ;
#8581=ORIENTED_EDGE ( 'NONE', *, *, #20182, .F. ) ;
#8584=CARTESIAN_POINT ( 'NONE',  ( -3.756430356249997882, 28.51562499938548711, 8.999999999999992895 ) ) ;
#8598=CYLINDRICAL_SURFACE ( 'NONE', #25825, 0.5000000000000004441 ) ;
#8604=CARTESIAN_POINT ( 'NONE',  ( 3.469446951953614189E-15, 31.50000000000000000, 8.999999999999992895 ) ) ;
#8607=CARTESIAN_POINT ( 'NONE',  ( 3.469446951953614189E-15, 25.00000000000000000, 8.999999999999992895 ) ) ;
#8621=( LENGTH_UNIT ( ) NAMED_UNIT ( * ) SI_UNIT ( .MILLI., .METRE. ) );
#8637=DIRECTION ( 'NONE',  ( 0.000000000000000000, 0.000000000000000000, -1.000000000000000000 ) ) ;
#8659=CARTESIAN_POINT ( 'NONE',  ( 3.253724281355068545E-15, 25.50624999877097210, 4.999999999999992006 ) ) ;
#8664=CARTESIAN_POINT ( 'NONE',  ( 0.000000000000000000, 28.74062499938548854, 13.33755215474602984 ) ) ;
#8667=DIRECTION ( 'NONE',  ( -0.000000000000000000, 1.000000000000000000, -0.000000000000000000 ) ) ;
#8669=CARTESIAN_POINT ( 'NONE',  ( 5.532151103383234236, 31.50000000000000000, 6.677220593914319657 ) ) ;
#8675=CARTESIAN_POINT ( 'NONE',  ( -0.4553717634079568755, 38.72245023127407393, 14.76006188199138869 ) ) ;
#8680=CARTESIAN_POINT ( 'NONE',  ( -3.999999999999998224, 29.27500000000000568, 8.999999999999992895 ) ) ;
#8682=DIRECTION ( 'NONE',  ( 0.000000000000000000, 0.000000000000000000, 1.000000000000000000 ) ) ;
#8685=CARTESIAN_POINT ( 'NONE',  ( 3.469446951953614189E-15, 38.49999999999999289, 8.999999999999992895 ) ) ;
#8704=CARTESIAN_POINT ( 'NONE',  ( 4.000000000000001776, 26.35000000000000497, 8.999999999999992895 ) ) ;
#8705=CARTESIAN_POINT ( 'NONE',  ( 0.000000000000000000, 25.92812499938548854, 13.33755215474602984 ) ) ;
#8711=CARTESIAN_POINT ( 'NONE',  ( 3.959305671612554781E-15, 35.50000000000000711, 12.99999999999999289 ) ) ;
#8721=CARTESIAN_POINT ( 'NONE',  ( -1.071796769724487230, 25.52634618820331269, 4.999999999999992895 ) ) ;
#8731=ORIENTED_EDGE ( 'NONE', *, *, #5020, .F. ) ;
#8738=CARTESIAN_POINT ( 'NONE',  ( -2.003086131649545506E-15, 26.04062499938549280, 13.33755215474602984 ) ) ;
#8757=CYLINDRICAL_SURFACE ( 'NONE', #9547, 4.000000000000000000 ) ;
#8764=ORIENTED_EDGE ( 'NONE', *, *, #144, .F. ) ;
#8767=VECTOR ( 'NONE', #19376, 1000.000000000000000 ) ;
#8768=VERTEX_POINT ( 'NONE', #11225 ) ;
#8770=ORIENTED_EDGE ( 'NONE', *, *, #5089, .F. ) ;
#8771=ADVANCED_FACE ( 'NONE', ( #15042 ), #17135, .F. ) ;
#8775=ORIENTED_EDGE ( 'NONE', *, *, #22800, .T. ) ;
#8798=CARTESIAN_POINT ( 'NONE',  ( 1.878215178125001605, 28.77812499938549351, 12.25316411605952283 ) ) ;
#8805=CARTESIAN_POINT ( 'NONE',  ( -1.999999999999994893, 27.79374999877096997, 5.535898384862237620 ) ) ;
#8815=CARTESIAN_POINT ( 'NONE',  ( 3.959305671612554781E-15, 35.50000000000000711, 12.99999999999999289 ) ) ;
#8827=CARTESIAN_POINT ( 'NONE',  ( -3.999999999999996447, 26.51874999877097494, 8.999999999999992895 ) ) ;
#8844=CARTESIAN_POINT ( 'NONE',  ( -3.756430356249996549, 26.71562499938548996, 8.999999999999992895 ) ) ;
#8846=CARTESIAN_POINT ( 'NONE',  ( 7.901901826148023498E-15, 26.23750000000000426, 12.99999999999999112 ) ) ;
#8847=CARTESIAN_POINT ( 'NONE',  ( 4.000000000000005329, 25.41250000000000497, 11.30940107675849760 ) ) ;
#8868=CARTESIAN_POINT ( 'NONE',  ( -1.071796769724487453, 25.71115380933864003, 12.99999999999999467 ) ) ;
#8876=AXIS2_PLACEMENT_3D ( 'NONE', #24284, #15928, #20219 ) ;
#8884=CARTESIAN_POINT ( 'NONE',  ( 3.756430356250003211, 28.40312499938548640, 8.999999999999992895 ) ) ;
#8903=ADVANCED_FACE ( 'NONE', ( #3909, #19967 ), #19730, .F. ) ;
#8924=CYLINDRICAL_SURFACE ( 'NONE', #10018, 4.000000000000000000 ) ;
#8932=CARTESIAN_POINT ( 'NONE',  ( -5.796869523101029209, 38.54567717719766762, 7.639754566698839788 ) ) ;
#8933=EDGE_CURVE ( 'NONE', #13400, #4609, #14445, .T. ) ;
#8963=CARTESIAN_POINT ( 'NONE',  ( 8.012344526598182026E-15, 28.65624999877097778, 4.381197846482986158 ) ) ;
#8969=CARTESIAN_POINT ( 'NONE',  ( 3.756430356250003211, 29.30312499938548498, 8.999999999999992895 ) ) ;
#8979=CARTESIAN_POINT ( 'NONE',  ( 6.009258394948636914E-15, 26.15312499938548640, 4.662447845253954171 ) ) ;
#8980=DIRECTION ( 'NONE',  ( 0.000000000000000000, 1.000000000000000000, 0.000000000000000000 ) ) ;
#8981=CARTESIAN_POINT ( 'NONE',  ( 2.000000000000000000, 25.37500000000000355, 12.46410161513774817 ) ) ;
#8982=CARTESIAN_POINT ( 'NONE',  ( 1.071796769724491671, 28.90134618820330559, 12.99999999999999467 ) ) ;
#8991=CARTESIAN_POINT ( 'NONE',  ( -3.110308778861381462, 34.50000000000000000, 3.869115154270378110 ) ) ;
#9000=EDGE_CURVE ( 'NONE', #15395, #12207, #25870, .T. ) ;
#9007=CARTESIAN_POINT ( 'NONE',  ( -3.756430356250000546, 28.21562499938548640, 11.16877607737301226 ) ) ;
#9010=CARTESIAN_POINT ( 'NONE',  ( -3.027295627619581708, 38.86045373840903494, 4.241260441470868336 ) ) ;
#9013=LINE ( 'NONE', #12936, #11713 ) ;
#9023=ORIENTED_EDGE ( 'NONE', *, *, #11186, .T. ) ;
#9024=DIRECTION ( 'NONE',  ( 0.000000000000000000, -1.000000000000000000, 0.000000000000000000 ) ) ;
#9058=ORIENTED_EDGE ( 'NONE', *, *, #25170, .F. ) ;
#9059=CARTESIAN_POINT ( 'NONE',  ( -1.071796769724482123, 27.96115380933863648, 12.99999999999999645 ) ) ;
#9069=CYLINDRICAL_SURFACE ( 'NONE', #10026, 4.000000000000000000 ) ;
#9076=CARTESIAN_POINT ( 'NONE',  ( -3.999999999999999556, 28.35624999877097707, 11.30940107675849404 ) ) ;
#9091=CARTESIAN_POINT ( 'NONE',  ( 3.756430356250006319, 28.77812499938548640, 6.831223922626973533 ) ) ;
#9099=CARTESIAN_POINT ( 'NONE',  ( -5.706339097770935176, 29.50000000000000000, 7.645898033750358813 ) ) ;
#9117=ORIENTED_EDGE ( 'NONE', *, *, #1174, .F. ) ;
#9119=CARTESIAN_POINT ( 'NONE',  ( 1.878215178124999829, 28.32812499938549422, 12.25316411605952283 ) ) ;
#9147=CARTESIAN_POINT ( 'NONE',  ( 3.526711513754847704, 31.50000000000000000, 13.85410196624967405 ) ) ;
#9155=ORIENTED_EDGE ( 'NONE', *, *, #2241, .F. ) ;
#9184=VECTOR ( 'NONE', #21151, 1000.000000000000000 ) ;
#9211=CARTESIAN_POINT ( 'NONE',  ( 6.009258394948636914E-15, 27.75624999877097920, 4.381197846482986158 ) ) ;
#9219=ORIENTED_EDGE ( 'NONE', *, *, #7590, .F. ) ;
#9227=CARTESIAN_POINT ( 'NONE',  ( 3.756430356250004987, 29.64062499938548711, 8.999999999999992895 ) ) ;
#9228=CARTESIAN_POINT ( 'NONE',  ( 1.878215178125001605, 26.41562499938548925, 12.25316411605952283 ) ) ;
#9231=CARTESIAN_POINT ( 'NONE',  ( 1.878215178125001605, 29.11562499938549209, 12.25316411605952283 ) ) ;
#9233=AXIS2_PLACEMENT_3D ( 'NONE', #4239, #20186, #12466 ) ;
#9248=CARTESIAN_POINT ( 'NONE',  ( -1.394453263437886604E-15, 27.30624999877096926, 4.999999999999991118 ) ) ;
#9250=CARTESIAN_POINT ( 'NONE',  ( -1.859271017917182139E-15, 26.46249999999999858, 4.999999999999991118 ) ) ;
#9258=EDGE_CURVE ( 'NONE', #18497, #1729, #15147, .T. ) ;
#9263=DIRECTION ( 'NONE',  ( 0.000000000000000000, 1.000000000000000000, 0.000000000000000000 ) ) ;
#9265=CARTESIAN_POINT ( 'NONE',  ( 3.756430356250004543, 27.01562499938549067, 11.16877607737301226 ) ) ;
#9271=CARTESIAN_POINT ( 'NONE',  ( 6.938893903907228378E-15, 29.50000000000000000, 2.999999999999992450 ) ) ;
#9281=CIRCLE ( 'NONE', #4689, 5.000000000000000888 ) ;
#9287=ORIENTED_EDGE ( 'NONE', *, *, #18776, .T. ) ;
#9301=CARTESIAN_POINT ( 'NONE',  ( 3.756430356250004987, 25.14062499938548356, 8.999999999999992895 ) ) ;
#9311=LINE ( 'NONE', #7343, #17625 ) ;
#9321=VERTEX_POINT ( 'NONE', #9250 ) ;
#9328=DIRECTION ( 'NONE',  ( 0.000000000000000000, 0.000000000000000000, -1.000000000000000000 ) ) ;
#9332=ADVANCED_FACE ( 'NONE', ( #23737 ), #19691, .T. ) ;
#9339=DIRECTION ( 'NONE',  ( 0.000000000000000000, 0.000000000000000000, 1.000000000000000000 ) ) ;
#9343=EDGE_CURVE ( 'NONE', #345, #23841, #24956, .T. ) ;
#9347=CARTESIAN_POINT ( 'NONE',  ( 4.000000000000001776, 27.19374999877097210, 8.999999999999992895 ) ) ;
#9357=CARTESIAN_POINT ( 'NONE',  ( 3.718542035834364277E-15, 25.11250000000000782, 4.999999999999992006 ) ) ;
#9361=CARTESIAN_POINT ( 'NONE',  ( 6.009258394948636914E-15, 27.95312499938548356, 4.662447845253954171 ) ) ;
#9363=CARTESIAN_POINT ( 'NONE',  ( -3.756430356249997882, 29.41562499938548569, 8.999999999999992895 ) ) ;
#9365=EDGE_CURVE ( 'NONE', #1139, #11943, #10439, .T. ) ;
#9392=CARTESIAN_POINT ( 'NONE',  ( 3.756430356250006319, 25.17812499938548854, 6.831223922626973533 ) ) ;
#9411=ORIENTED_EDGE ( 'NONE', *, *, #4873, .T. ) ;
#9422=CARTESIAN_POINT ( 'NONE',  ( -3.756430356249996105, 25.32812499938549067, 6.831223922626973533 ) ) ;
#9442=ORIENTED_EDGE ( 'NONE', *, *, #9343, .F. ) ;
#9453=CARTESIAN_POINT ( 'NONE',  ( -3.918623196469520842, 31.50000000000000000, 4.456389954662587805 ) ) ;
#9460=EDGE_CURVE ( 'NONE', #2153, #22574, #16315, .T. ) ;
#9466=CARTESIAN_POINT ( 'NONE',  ( 6.009258394948636914E-15, 27.30624999877097636, 4.381197846482986158 ) ) ;
#9478=CARTESIAN_POINT ( 'NONE',  ( -3.756430356249996549, 27.65312499938548996, 11.16877607737301048 ) ) ;
#9480=CARTESIAN_POINT ( 'NONE',  ( -3.999999999999998224, 27.02500000000000213, 8.999999999999992895 ) ) ;
#9485=CARTESIAN_POINT ( 'NONE',  ( -1.071796769724490783, 27.06115380933863790, 12.99999999999999289 ) ) ;
#9506=CARTESIAN_POINT ( 'NONE',  ( 3.110308778861350376, 34.50000000000000000, 14.13088484572963033 ) ) ;
#9507=CARTESIAN_POINT ( 'NONE',  ( 3.756430356250002323, 25.62812499938548072, 6.831223922626973533 ) ) ;
#9533=EDGE_LOOP ( 'NONE', ( #23783, #24370, #11015, #6513 ) ) ;
#9541=ADVANCED_FACE ( 'NONE', ( #1094 ), #9069, .T. ) ;
#9547=AXIS2_PLACEMENT_3D ( 'NONE', #23019, #7315, #24968 ) ;
#9571=VECTOR ( 'NONE', #25832, 1000.000000000000000 ) ;
#9572=ORIENTED_EDGE ( 'NONE', *, *, #23291, .F. ) ;
#9590=CARTESIAN_POINT ( 'NONE',  ( -1.999999999999994893, 29.14374999877097139, 5.535898384862237620 ) ) ;
#9599=EDGE_CURVE ( 'NONE', #7412, #486, #2734, .T. ) ;
#9606=CARTESIAN_POINT ( 'NONE',  ( 3.756430356250006319, 28.77812499938548640, 6.831223922626973533 ) ) ;
#9611=CARTESIAN_POINT ( 'NONE',  ( -3.999999999999999556, 26.61250000000000426, 11.30940107675849404 ) ) ;
#9628=CARTESIAN_POINT ( 'NONE',  ( 2.000000000000003553, 25.91874999877097352, 5.535898384862238508 ) ) ;
#9633=CARTESIAN_POINT ( 'NONE',  ( 2.003086131649545506E-15, 25.59062499938548996, 13.33755215474603162 ) ) ;
#9642=CARTESIAN_POINT ( 'NONE',  ( -3.756430356249996105, 25.40312499938548640, 11.16877607737301226 ) ) ;
#9648=SURFACE_STYLE_FILL_AREA ( #23248 ) ;
#9653=CARTESIAN_POINT ( 'NONE',  ( 2.000000000000000000, 28.97500000000000853, 12.46410161513774817 ) ) ;
#9666=DIRECTION ( 'NONE',  ( 0.000000000000000000, 1.000000000000000000, 0.000000000000000000 ) ) ;
#9681=CARTESIAN_POINT ( 'NONE',  ( -3.999999999999994671, 27.88750000000000639, 6.690598923241487306 ) ) ;
#9712=AXIS2_PLACEMENT_3D ( 'NONE', #9271, #13193, #21164 ) ;
#9723=CARTESIAN_POINT ( 'NONE',  ( -9.296355089585909904E-15, 29.10624999877097352, 4.999999999999992006 ) ) ;
#9731=CARTESIAN_POINT ( 'NONE',  ( 1.878215178125005158, 25.77812499938548996, 5.746835883940462963 ) ) ;
#9741=CARTESIAN_POINT ( 'NONE',  ( 3.100771756283734248, 38.96317070936194682, 4.412623259661243580 ) ) ;
#9743=CARTESIAN_POINT ( 'NONE',  ( 4.006172263299091013E-15, 28.40312499938548996, 4.662447845253954171 ) ) ;
#9745=CARTESIAN_POINT ( 'NONE',  ( -1.999999999999994893, 27.85000000000000497, 5.535898384862237620 ) ) ;
#9763=CARTESIAN_POINT ( 'NONE',  ( -3.756430356249996549, 25.47812499938548925, 8.999999999999992895 ) ) ;
#9774=CARTESIAN_POINT ( 'NONE',  ( -3.756430356249994773, 25.81562499938548783, 8.999999999999992895 ) ) ;
#9784=ORIENTED_EDGE ( 'NONE', *, *, #11186, .F. ) ;
#9785=CARTESIAN_POINT ( 'NONE',  ( -5.532151103383211144, 38.49999999999999289, 11.32277940608570255 ) ) ;
#9795=CARTESIAN_POINT ( 'NONE',  ( 4.000000000000003553, 28.54374999877097707, 8.999999999999992895 ) ) ;
#9806=CARTESIAN_POINT ( 'NONE',  ( -2.003086131649545506E-15, 27.27812499938548640, 13.33755215474602984 ) ) ;
#9837=DIRECTION ( 'NONE',  ( 0.000000000000000000, 0.000000000000000000, -1.000000000000000000 ) ) ;
#9844=DIRECTION ( 'NONE',  ( 0.000000000000000000, 0.000000000000000000, -1.000000000000000000 ) ) ;
#9850=CARTESIAN_POINT ( 'NONE',  ( -3.756430356249998326, 25.51562499938549067, 11.16877607737301226 ) ) ;
#9851=EDGE_LOOP ( 'NONE', ( #305, #6351, #20244, #15774 ) ) ;
#9864=CARTESIAN_POINT ( 'NONE',  ( 1.878215178125003382, 28.36562499938548498, 5.746835883940462963 ) ) ;
#9866=CARTESIAN_POINT ( 'NONE',  ( 2.000000000000005329, 27.77500000000000568, 5.535898384862238508 ) ) ;
#9867=EDGE_CURVE ( 'NONE', #4609, #2753, #24668, .T. ) ;
#9877=CARTESIAN_POINT ( 'NONE',  ( 1.071796769724495446, 25.93615380933863790, 4.999999999999992895 ) ) ;
#9888=ORIENTED_EDGE ( 'NONE', *, *, #5167, .F. ) ;
#9890=CARTESIAN_POINT ( 'NONE',  ( -1.878215178124998275, 25.89062499938549067, 12.25316411605951927 ) ) ;
#9900=CARTESIAN_POINT ( 'NONE',  ( 3.469446951953614189E-15, 31.50000000000000000, 8.999999999999992895 ) ) ;
#9904=CARTESIAN_POINT ( 'NONE',  ( 5.606326150107658890, 38.73250905386370135, 7.645898033760625268 ) ) ;
#9922=CARTESIAN_POINT ( 'NONE',  ( 1.878215178125001605, 27.31562499938548783, 12.25316411605952283 ) ) ;
#9933=CYLINDRICAL_SURFACE ( 'NONE', #17567, 4.000000000000000000 ) ;
#9943=ORIENTED_EDGE ( 'NONE', *, *, #6789, .T. ) ;
#9944=CARTESIAN_POINT ( 'NONE',  ( 7.437084071668728555E-15, 27.13750000000000639, 12.99999999999999112 ) ) ;
#9949=CIRCLE ( 'NONE', #7017, 0.5000000000000004441 ) ;
#9952=VERTEX_POINT ( 'NONE', #10444 ) ;
#9974=CARTESIAN_POINT ( 'NONE',  ( 3.756430356250003211, 25.70312499938548356, 8.999999999999992895 ) ) ;
#9984=CARTESIAN_POINT ( 'NONE',  ( 0.2827178117968801030, 38.91165577845126222, 14.58153869134143577 ) ) ;
#9987=CARTESIAN_POINT ( 'NONE',  ( 0.4949451094549379704, 38.61079987549954495, 3.131633208832877102 ) ) ;
#9989=CARTESIAN_POINT ( 'NONE',  ( 0.000000000000000000, 26.23750000000000426, 13.61880215351699874 ) ) ;
#9996=CIRCLE ( 'NONE', #22948, 6.000000000000000000 ) ;
#10001=EDGE_CURVE ( 'NONE', #13400, #15214, #10576, .T. ) ;
#10009=CARTESIAN_POINT ( 'NONE',  ( -3.756430356249996549, 26.82812499938549067, 8.999999999999992895 ) ) ;
#10017=CARTESIAN_POINT ( 'NONE',  ( -3.756430356249996105, 28.92812499938548498, 6.831223922626973533 ) ) ;
#10018=AXIS2_PLACEMENT_3D ( 'NONE', #10606, #4594, #12714 ) ;
#10026=AXIS2_PLACEMENT_3D ( 'NONE', #1363, #17052, #25023 ) ;
#10027=DIRECTION ( 'NONE',  ( 0.000000000000000000, 1.000000000000000000, 0.000000000000000000 ) ) ;
#10034=CARTESIAN_POINT ( 'NONE',  ( -5.221103800765325431, 38.91143067427094593, 10.99401152278178451 ) ) ;
#10056=CARTESIAN_POINT ( 'NONE',  ( 3.756430356250002323, 26.45312499938549067, 11.16877607737301226 ) ) ;
#10060=( BOUNDED_SURFACE ( )  B_SPLINE_SURFACE ( 1, 2, ( 
 ( #10181, #6262, #22472, #12403, #12146, #765, #10568, #20511, #386, #8356, #24556, #10432, #14252, #22222, #525, #22613, #16480, #4308, #10692, #12281, #18565, #8738, #4552, #6644, #24048, #2346, #6130, #14116, #22079, #20122, #20247, #16345, #24312, #6397, #14387, #22345, #11203, #13310, #13064, #19325, #21043, #6909, #10818, #21283, #3118, #3365, #11083, #9265, #19064, #1147, #24699, #4822, #25085, #16986, #5328, #11342, #1419, #23245, #16725, #6785, #14770, #19183, #24950, #7030, #22746, #16867, #12926, #1280, #2991, #13189, #12799, #4941, #15018, #20773, #3232, #2851, #18812, #24833, #902, #9007, #17253, #21159, #9119, #17110, #8884, #7173, #14891, #22865, #25221, #20902, #10961, #18947, #7301, #15161, #22998, #1031, #5084, #23129, #5212, #15280, #11591, #13827, #15920, #17624, #11729, #11474, #21540, #15782, #3748, #17372, #15397, #11975, #21804, #23751, #3621, #19564, #11859, #5710, #1538, #19444, #15666 ),
 ( #1668, #9392, #25339, #13453, #19827, #7803, #21421, #9642, #5594, #13574, #19705, #23507, #7417, #9507, #1806, #3502, #21929, #23374, #9774, #17487, #9890, #5459, #25461, #17750, #7547, #13689, #23895, #25598, #23633, #15541, #7681, #21663, #25722, #5840, #3885, #1928, #17876, #25847, #7933, #5976, #13958, #4009, #19947, #12109, #22437, #20085, #6362, #6098, #2566, #22314, #14352, #20213, #24016, #18262, #22576, #2313, #4130, #22046, #6486, #101, #2428, #14472, #12493, #4515, #18390, #20469, #18013, #4392, #6606, #12372, #10390, #2187, #618, #14081, #10148, #8074, #10268, #18152, #16053, #224, #10534, #14592, #20336, #8195, #18532, #16171, #488, #24136, #6221, #16446, #8584, #8459, #16564, #24524, #8318, #14213, #12638, #4656, #2050, #22186, #24411, #10017, #4273, #12244, #348, #16306, #24274, #19152, #11169, #25047, #15123, #18772, #5045, #22711, #13027, #23212, #5296, #21122, #10779, #4792, #9227 ) ),
 .UNSPECIFIED., .F., .F., .F. ) 
 B_SPLINE_SURFACE_WITH_KNOTS ( ( 2, 2 ),
 ( 3, 2, 2, 2, 2, 2, 2, 2, 2, 2, 2, 2, 2, 2, 2, 2, 2, 2, 2, 2, 2, 2, 2, 2, 2, 2, 2, 2, 2, 2, 2, 2, 2, 2, 2, 2, 2, 2, 2, 2, 2, 2, 2, 2, 2, 2, 2, 2, 2, 2, 2, 2, 2, 2, 2, 2, 2, 2, 2, 2, 3 ),
 ( 0.000000000000000000, 1.000000000000000000 ),
 ( 0.000000000000000000, 0.01666666666666666644, 0.03333333333333333287, 0.05000000000000000278, 0.06666666666666666574, 0.08333333333333332871, 0.1000000000000000056, 0.1166666666666666685, 0.1333333333333333315, 0.1499999999999999944, 0.1666666666666666574, 0.1833333333333333204, 0.2000000000000000111, 0.2166666666666666741, 0.2333333333333333370, 0.2500000000000000000, 0.2666666666666666630, 0.2833333333333333259, 0.2999999999999999889, 0.3166666666666666519, 0.3333333333333333148, 0.3499999999999999778, 0.3666666666666666408, 0.3833333333333333592, 0.4000000000000000222, 0.4166666666666666852, 0.4333333333333333481, 0.4500000000000000111, 0.4666666666666666741, 0.4833333333333333370, 0.5000000000000000000, 0.5166666666666667185, 0.5333333333333333259, 0.5500000000000000444, 0.5666666666666666519, 0.5833333333333333703, 0.5999999999999999778, 0.6166666666666666963, 0.6333333333333333037, 0.6500000000000000222, 0.6666666666666666297, 0.6833333333333333481, 0.6999999999999999556, 0.7166666666666666741, 0.7333333333333332815, 0.7500000000000000000, 0.7666666666666667185, 0.7833333333333333259, 0.8000000000000000444, 0.8166666666666666519, 0.8333333333333333703, 0.8499999999999999778, 0.8666666666666666963, 0.8833333333333333037, 0.9000000000000000222, 0.9166666666666666297, 0.9333333333333333481, 0.9499999999999999556, 0.9666666666666666741, 0.9833333333333332815, 1.000000000000000000 ),
 .UNSPECIFIED. ) 
 GEOMETRIC_REPRESENTATION_ITEM ( )  RATIONAL_B_SPLINE_SURFACE ( (
 ( 1.000000000000000000, 0.8660254037844387076, 1.000000000000000000, 0.8660254037844387076, 1.000000000000000000, 0.8660254037844387076, 1.000000000000000000, 0.8660254037844387076, 1.000000000000000000, 0.8660254037844387076, 1.000000000000000000, 0.8660254037844387076, 1.000000000000000000, 0.8660254037844387076, 1.000000000000000000, 0.8660254037844387076, 1.000000000000000000, 0.8660254037844387076, 1.000000000000000000, 0.8660254037844387076, 1.000000000000000000, 0.8660254037844387076, 1.000000000000000000, 0.8660254037844387076, 1.000000000000000000, 0.8660254037844387076, 1.000000000000000000, 0.8660254037844387076, 1.000000000000000000, 0.8660254037844387076, 1.000000000000000000, 0.8660254037844387076, 1.000000000000000000, 0.8660254037844387076, 1.000000000000000000, 0.8660254037844387076, 1.000000000000000000, 0.8660254037844387076, 1.000000000000000000, 0.8660254037844387076, 1.000000000000000000, 0.8660254037844387076, 1.000000000000000000, 0.8660254037844387076, 1.000000000000000000, 0.8660254037844387076, 1.000000000000000000, 0.8660254037844387076, 1.000000000000000000, 0.8660254037844387076, 1.000000000000000000, 0.8660254037844387076, 1.000000000000000000, 0.8660254037844387076, 1.000000000000000000, 0.8660254037844387076, 1.000000000000000000, 0.8660254037844387076, 1.000000000000000000, 0.8660254037844387076, 1.000000000000000000, 0.8660254037844387076, 1.000000000000000000, 0.8660254037844387076, 1.000000000000000000, 0.8660254037844387076, 1.000000000000000000, 0.8660254037844387076, 1.000000000000000000, 0.8660254037844387076, 1.000000000000000000, 0.8660254037844387076, 1.000000000000000000, 0.8660254037844387076, 1.000000000000000000, 0.8660254037844387076, 1.000000000000000000, 0.8660254037844387076, 1.000000000000000000, 0.8660254037844387076, 1.000000000000000000, 0.8660254037844387076, 1.000000000000000000, 0.8660254037844387076, 1.000000000000000000, 0.8660254037844387076, 1.000000000000000000, 0.8660254037844387076, 1.000000000000000000, 0.8660254037844387076, 1.000000000000000000, 0.8660254037844387076, 1.000000000000000000, 0.8660254037844387076, 1.000000000000000000, 0.8660254037844387076, 1.000000000000000000, 0.8660254037844387076, 1.000000000000000000, 0.8660254037844387076, 1.000000000000000000, 0.8660254037844387076, 1.000000000000000000, 0.8660254037844387076, 1.000000000000000000, 0.8660254037844387076, 1.000000000000000000, 0.8660254037844387076, 1.000000000000000000, 0.8660254037844387076, 1.000000000000000000, 0.8660254037844387076, 1.000000000000000000, 0.8660254037844387076, 1.000000000000000000, 0.8660254037844387076, 1.000000000000000000, 0.8660254037844387076, 1.000000000000000000, 0.8660254037844387076, 1.000000000000000000),
 ( 1.000000000000000000, 0.8660254037844387076, 1.000000000000000000, 0.8660254037844387076, 1.000000000000000000, 0.8660254037844387076, 1.000000000000000000, 0.8660254037844387076, 1.000000000000000000, 0.8660254037844387076, 1.000000000000000000, 0.8660254037844387076, 1.000000000000000000, 0.8660254037844387076, 1.000000000000000000, 0.8660254037844387076, 1.000000000000000000, 0.8660254037844387076, 1.000000000000000000, 0.8660254037844387076, 1.000000000000000000, 0.8660254037844387076, 1.000000000000000000, 0.8660254037844387076, 1.000000000000000000, 0.8660254037844387076, 1.000000000000000000, 0.8660254037844387076, 1.000000000000000000, 0.8660254037844387076, 1.000000000000000000, 0.8660254037844387076, 1.000000000000000000, 0.8660254037844387076, 1.000000000000000000, 0.8660254037844387076, 1.000000000000000000, 0.8660254037844387076, 1.000000000000000000, 0.8660254037844387076, 1.000000000000000000, 0.8660254037844387076, 1.000000000000000000, 0.8660254037844387076, 1.000000000000000000, 0.8660254037844387076, 1.000000000000000000, 0.8660254037844387076, 1.000000000000000000, 0.8660254037844387076, 1.000000000000000000, 0.8660254037844387076, 1.000000000000000000, 0.8660254037844387076, 1.000000000000000000, 0.8660254037844387076, 1.000000000000000000, 0.8660254037844387076, 1.000000000000000000, 0.8660254037844387076, 1.000000000000000000, 0.8660254037844387076, 1.000000000000000000, 0.8660254037844387076, 1.000000000000000000, 0.8660254037844387076, 1.000000000000000000, 0.8660254037844387076, 1.000000000000000000, 0.8660254037844387076, 1.000000000000000000, 0.8660254037844387076, 1.000000000000000000, 0.8660254037844387076, 1.000000000000000000, 0.8660254037844387076, 1.000000000000000000, 0.8660254037844387076, 1.000000000000000000, 0.8660254037844387076, 1.000000000000000000, 0.8660254037844387076, 1.000000000000000000, 0.8660254037844387076, 1.000000000000000000, 0.8660254037844387076, 1.000000000000000000, 0.8660254037844387076, 1.000000000000000000, 0.8660254037844387076, 1.000000000000000000, 0.8660254037844387076, 1.000000000000000000, 0.8660254037844387076, 1.000000000000000000, 0.8660254037844387076, 1.000000000000000000, 0.8660254037844387076, 1.000000000000000000, 0.8660254037844387076, 1.000000000000000000, 0.8660254037844387076, 1.000000000000000000, 0.8660254037844387076, 1.000000000000000000, 0.8660254037844387076, 1.000000000000000000, 0.8660254037844387076, 1.000000000000000000, 0.8660254037844387076, 1.000000000000000000, 0.8660254037844387076, 1.000000000000000000, 0.8660254037844387076, 1.000000000000000000, 0.8660254037844387076, 1.000000000000000000, 0.8660254037844387076, 1.000000000000000000, 0.8660254037844387076, 1.000000000000000000) ) ) 
 REPRESENTATION_ITEM ( '' )  SURFACE ( )  );
#10063=VECTOR ( 'NONE', #10756, 1000.000000000000000 ) ;
#10069=AXIS2_PLACEMENT_3D ( 'NONE', #19303, #13172, #21022 ) ;
#10073=CARTESIAN_POINT ( 'NONE',  ( 4.000000000000002665, 28.13124999877096855, 6.690598923241489970 ) ) ;
#10076=CARTESIAN_POINT ( 'NONE',  ( -3.999999999999994671, 26.98750000000000426, 6.690598923241487306 ) ) ;
#10095=FACE_OUTER_BOUND ( 'NONE', #9533, .T. ) ;
#10103=CARTESIAN_POINT ( 'NONE',  ( 4.000000000000003553, 28.15000000000000924, 8.999999999999992895 ) ) ;
#10104=VERTEX_POINT ( 'NONE', #6795 ) ;
#10106=CARTESIAN_POINT ( 'NONE',  ( 0.000000000000000000, 29.33124999877097139, 13.61880215351699874 ) ) ;
#10109=EDGE_CURVE ( 'NONE', #11133, #1139, #9013, .T. ) ;
#10113=CARTESIAN_POINT ( 'NONE',  ( -1.022599059854450137E-14, 29.16250000000000497, 4.999999999999992006 ) ) ;
#10115=CARTESIAN_POINT ( 'NONE',  ( 4.648177544792955347E-16, 28.48750000000000071, 12.99999999999999289 ) ) ;
#10124=CARTESIAN_POINT ( 'NONE',  ( 1.878215178125003382, 29.56562499938549138, 12.25316411605952283 ) ) ;
#10131=CYLINDRICAL_SURFACE ( 'NONE', #6380, 0.5000000000000004441 ) ;
#10139=CARTESIAN_POINT ( 'NONE',  ( -3.756430356249994773, 26.37812499938548783, 8.999999999999992895 ) ) ;
#10140=ORIENTED_EDGE ( 'NONE', *, *, #24866, .F. ) ;
#10142=CARTESIAN_POINT ( 'NONE',  ( 3.918623196469464443, 38.49999999999999289, 4.456389954662531849 ) ) ;
#10148=CARTESIAN_POINT ( 'NONE',  ( 1.878215178125006934, 27.91562499938549280, 5.746835883940462963 ) ) ;
#10161=CARTESIAN_POINT ( 'NONE',  ( -3.999999999999996447, 26.48124999877096997, 6.690598923241487306 ) ) ;
#10181=CARTESIAN_POINT ( 'NONE',  ( 3.756430356250004987, 25.25312499938548427, 8.999999999999992895 ) ) ;
#10183=CARTESIAN_POINT ( 'NONE',  ( 3.756430356250006319, 26.97812499938548569, 6.831223922626973533 ) ) ;
#10189=DIRECTION ( 'NONE',  ( -0.000000000000000000, -1.000000000000000000, -0.000000000000000000 ) ) ;
#10207=CARTESIAN_POINT ( 'NONE',  ( 5.840899737312979845, 38.49999999999999289, 10.37254881831474052 ) ) ;
#10212=AXIS2_PLACEMENT_3D ( 'NONE', #1382, #5293, #15244 ) ;
#10228=CARTESIAN_POINT ( 'NONE',  ( 1.878215178124999829, 26.97812499938549280, 12.25316411605952283 ) ) ;
#10239=CARTESIAN_POINT ( 'NONE',  ( -3.756430356249997882, 29.41562499938548569, 8.999999999999992895 ) ) ;
#10259=CARTESIAN_POINT ( 'NONE',  ( 8.012344526598182026E-15, 28.06562499938548783, 4.662447845253954171 ) ) ;
#10263=CARTESIAN_POINT ( 'NONE',  ( 2.000000000000000000, 27.17500000000000426, 12.46410161513774817 ) ) ;
#10268=CARTESIAN_POINT ( 'NONE',  ( -1.878215178124994722, 27.99062499938548143, 5.746835883940462963 ) ) ;
#10301=B_SPLINE_CURVE_WITH_KNOTS ( 'NONE', 3,
 ( #13929, #19799, #13791, #2016, #25424, #23471, #9984, #5560, #17977, #7647 ),
 .UNSPECIFIED., .F., .F.,
 ( 4, 2, 2, 2, 4 ),
 ( 2.789812635319129240E-07, 0.0002324414413947202324, 0.0004646039015259085148, 0.0006967663616570968785, 0.0009289288217882851880 ),
 .UNSPECIFIED. ) ;
#10309=EDGE_CURVE ( 'NONE', #18698, #9952, #4142, .T. ) ;
#10330=ORIENTED_EDGE ( 'NONE', *, *, #5087, .T. ) ;
#10334=CARTESIAN_POINT ( 'NONE',  ( 5.112995299272250684E-15, 26.01250000000000284, 4.999999999999992006 ) ) ;
#10345=ORIENTED_EDGE ( 'NONE', *, *, #2480, .F. ) ;
#10346=CARTESIAN_POINT ( 'NONE',  ( 1.878215178125001605, 27.42812499938548854, 12.25316411605952283 ) ) ;
#10348=ORIENTED_EDGE ( 'NONE', *, *, #23410, .F. ) ;
#10363=DIRECTION ( 'NONE',  ( 0.000000000000000000, 0.000000000000000000, -1.000000000000000000 ) ) ;
#10364=CARTESIAN_POINT ( 'NONE',  ( -3.999999999999996447, 28.78750000000000497, 6.690598923241487306 ) ) ;
#10375=LINE ( 'NONE', #4378, #15020 ) ;
#10379=CARTESIAN_POINT ( 'NONE',  ( 3.756430356250002323, 28.44062499938548783, 6.831223922626973533 ) ) ;
#10390=CARTESIAN_POINT ( 'NONE',  ( 1.878215178125001605, 27.76562499938548711, 12.25316411605952283 ) ) ;
#10394=EDGE_CURVE ( 'NONE', #4893, #19796, #8234, .T. ) ;
#10402=CARTESIAN_POINT ( 'NONE',  ( -1.999999999999996669, 26.59374999877097423, 12.46410161513774639 ) ) ;
#10411=VERTEX_POINT ( 'NONE', #23640 ) ;
#10420=EDGE_LOOP ( 'NONE', ( #24466, #8775, #2248, #8573 ) ) ;
#10432=CARTESIAN_POINT ( 'NONE',  ( 3.756430356250002323, 25.66562499938548925, 11.16877607737301226 ) ) ;
#10439=CIRCLE ( 'NONE', #7529, 0.5000000000000004441 ) ;
#10444=CARTESIAN_POINT ( 'NONE',  ( 3.469446951953614189E-15, 25.00000000000000000, 4.999999999999992006 ) ) ;
#10446=FACE_OUTER_BOUND ( 'NONE', #11043, .T. ) ;
#10450=CARTESIAN_POINT ( 'NONE',  ( 1.580380365229604700E-14, 27.58750000000000213, 12.99999999999999289 ) ) ;
#10461=ORIENTED_EDGE ( 'NONE', *, *, #1035, .F. ) ;
#10463=ORIENTED_EDGE ( 'NONE', *, *, #9599, .T. ) ;
#10479=CARTESIAN_POINT ( 'NONE',  ( 3.469446951953614189E-15, 35.50000000000000711, 8.999999999999992895 ) ) ;
#10482=CARTESIAN_POINT ( 'NONE',  ( -3.999999999999994671, 28.73124999877097352, 6.690598923241487306 ) ) ;
#10490=CARTESIAN_POINT ( 'NONE',  ( 8.012344526598182026E-15, 28.51562499938549067, 4.662447845253954171 ) ) ;
#10493=CYLINDRICAL_SURFACE ( 'NONE', #10840, 4.000000000000000000 ) ;
#10496=ORIENTED_EDGE ( 'NONE', *, *, #8933, .F. ) ;
#10497=CARTESIAN_POINT ( 'NONE',  ( -4.000000000000000000, 27.86874999877096926, 8.999999999999992895 ) ) ;
#10511=VECTOR ( 'NONE', #17535, 1000.000000000000000 ) ;
#10517=CARTESIAN_POINT ( 'NONE',  ( -3.999999999999996447, 25.65624999877097423, 11.30940107675849404 ) ) ;
#10525=CARTESIAN_POINT ( 'NONE',  ( 1.878215178125005158, 27.12812499938548783, 5.746835883940462963 ) ) ;
#10534=CARTESIAN_POINT ( 'NONE',  ( -1.878215178124998275, 28.14062499938548711, 12.25316411605951927 ) ) ;
#10550=AXIS2_PLACEMENT_3D ( 'NONE', #13085, #23022, #5107 ) ;
#10553=CARTESIAN_POINT ( 'NONE',  ( -1.999999999999996669, 25.69374999877097920, 12.46410161513774639 ) ) ;
#10555=EDGE_LOOP ( 'NONE', ( #6096, #12056, #15752, #4842, #13019, #23272, #8553, #12387, #20392, #16338, #7358, #21925, #6896, #15013, #20240, #12213, #16584, #1082, #11532, #2519, #7577, #24616, #16080, #4615 ) ) ;
#10556=DIRECTION ( 'NONE',  ( 0.000000000000000000, 1.000000000000000000, 0.000000000000000000 ) ) ;
#10568=CARTESIAN_POINT ( 'NONE',  ( -3.756430356249996549, 25.47812499938548925, 8.999999999999992895 ) ) ;
#10576=LINE ( 'NONE', #20780, #19664 ) ;
#10579=CARTESIAN_POINT ( 'NONE',  ( 3.878215178125005380, 25.32343749907823138, 8.999999999999992895 ) ) ;
#10593=( BOUNDED_CURVE ( )  B_SPLINE_CURVE ( 2, ( #7875, #3090, #18918, #5302, #11057, #3205, #14987, #12894, #1879 ),
 .UNSPECIFIED., .F., .F. ) 
 B_SPLINE_CURVE_WITH_KNOTS ( ( 3, 2, 2, 2, 3 ),
 ( 0.07500000000000001110, 0.08333333333333332871, 0.1000000000000000056, 0.1166666666666666685, 0.1250000000000000000 ),
 .UNSPECIFIED. ) 
 CURVE ( )  GEOMETRIC_REPRESENTATION_ITEM ( )  RATIONAL_B_SPLINE_CURVE ( ( 0.9330127018922192983, 0.9330127018922194093, 1.000000000000000000, 0.8660254037844387076, 1.000000000000000000, 0.8660254037844387076, 1.000000000000000000, 0.9330127018922194093, 0.9330127018922194093 ) ) 
 REPRESENTATION_ITEM ( '' )  );
#10606=CARTESIAN_POINT ( 'NONE',  ( 3.469446951953614189E-15, 35.50000000000000711, 8.999999999999992895 ) ) ;
#10619=VERTEX_POINT ( 'NONE', #23608 ) ;
#10620=CARTESIAN_POINT ( 'NONE',  ( -3.756430356249996105, 27.69062499938548427, 6.831223922626973533 ) ) ;
#10630=CARTESIAN_POINT ( 'NONE',  ( -1.998723687422152831E-12, 39.00000000001113420, 14.49999999998978240 ) ) ;
#10639=CARTESIAN_POINT ( 'NONE',  ( -0.4150711328764303820, 38.77044187147116361, 3.285374590644589254 ) ) ;
#10645=ORIENTED_EDGE ( 'NONE', *, *, #18717, .F. ) ;
#10659=CARTESIAN_POINT ( 'NONE',  ( 1.878215178125001605, 26.41562499938548925, 12.25316411605952283 ) ) ;
#10664=CARTESIAN_POINT ( 'NONE',  ( 5.577813053751546416E-15, 25.95624999877097139, 4.999999999999992006 ) ) ;
#10673=CARTESIAN_POINT ( 'NONE',  ( 5.577813053751546416E-15, 28.20624999877096784, 4.999999999999992006 ) ) ;
#10679=DIRECTION ( 'NONE',  ( 0.000000000000000000, 0.000000000000000000, 1.000000000000000000 ) ) ;
#10685=EDGE_CURVE ( 'NONE', #19796, #12137, #24113, .T. ) ;
#10692=CARTESIAN_POINT ( 'NONE',  ( -3.756430356249997882, 25.92812499938548854, 8.999999999999992895 ) ) ;
#10696=CARTESIAN_POINT ( 'NONE',  ( -3.110308778861381462, 38.49999999999999289, 3.869115154270378554 ) ) ;
#10735=CARTESIAN_POINT ( 'NONE',  ( -1.071796769724491671, 29.57634618820330275, 4.999999999999995559 ) ) ;
#10739=EDGE_LOOP ( 'NONE', ( #23116, #7610, #18974, #19113 ) ) ;
#10742=CARTESIAN_POINT ( 'NONE',  ( -3.756430356249994773, 29.07812499938548711, 8.999999999999992895 ) ) ;
#10749=CARTESIAN_POINT ( 'NONE',  ( 1.533898589781675205E-14, 27.98124999877097352, 12.99999999999999289 ) ) ;
#10756=DIRECTION ( 'NONE',  ( -0.000000000000000000, -1.000000000000000000, -0.000000000000000000 ) ) ;
#10766=CARTESIAN_POINT ( 'NONE',  ( -1.999999999999996669, 26.14374999877097494, 12.46410161513774639 ) ) ;
#10772=CARTESIAN_POINT ( 'NONE',  ( 0.000000000000000000, 29.64062499938549422, 13.33755215474603162 ) ) ;
#10775=CARTESIAN_POINT ( 'NONE',  ( 4.648177544792954952E-15, 25.73124999877097707, 12.99999999999999289 ) ) ;
#10779=CARTESIAN_POINT ( 'NONE',  ( 1.878215178125003382, 29.56562499938549138, 12.25316411605952283 ) ) ;
#10780=CARTESIAN_POINT ( 'NONE',  ( 1.878215178125006934, 25.21562499938548996, 5.746835883940462963 ) ) ;
#10782=CARTESIAN_POINT ( 'NONE',  ( -1.999999999999993117, 25.60000000000000497, 5.535898384862237620 ) ) ;
#10787=CARTESIAN_POINT ( 'NONE',  ( 3.526711513754847704, 29.50000000000000000, 13.85410196624967405 ) ) ;
#10795=AXIS2_PLACEMENT_3D ( 'NONE', #1727, #15324, #13367 ) ;
#10800=CARTESIAN_POINT ( 'NONE',  ( -5.532151103383211144, 38.49999999999999289, 11.32277940608570255 ) ) ;
#10818=CARTESIAN_POINT ( 'NONE',  ( -3.756430356249996549, 26.82812499938549067, 8.999999999999992895 ) ) ;
#10823=CIRCLE ( 'NONE', #8329, 6.000000000000000000 ) ;
#10833=DIRECTION ( 'NONE',  ( 0.000000000000000000, 1.000000000000000000, 0.000000000000000000 ) ) ;
#10840=AXIS2_PLACEMENT_3D ( 'NONE', #8549, #18351, #4227 ) ;
#10853=( BOUNDED_CURVE ( )  B_SPLINE_CURVE ( 2, ( #8846, #20741, #18777, #4517, #8704, #18265, #22317, #866, #16834 ),
 .UNSPECIFIED., .F., .F. ) 
 B_SPLINE_CURVE_WITH_KNOTS ( ( 3, 2, 2, 2, 3 ),
 ( 0.2750000000000000222, 0.2833333333333333259, 0.2999999999999999889, 0.3166666666666666519, 0.3250000000000000111 ),
 .UNSPECIFIED. ) 
 CURVE ( )  GEOMETRIC_REPRESENTATION_ITEM ( )  RATIONAL_B_SPLINE_CURVE ( ( 0.9330127018922194093, 0.9330127018922196314, 1.000000000000000000, 0.8660254037844387076, 1.000000000000000000, 0.8660254037844387076, 1.000000000000000000, 0.9330127018922191873, 0.9330127018922194093 ) ) 
 REPRESENTATION_ITEM ( '' )  );
#10855=CARTESIAN_POINT ( 'NONE',  ( 4.000000000000003553, 25.19687499938548925, 8.999999999999992895 ) ) ;
#10857=VECTOR ( 'NONE', #5367, 1000.000000000000000 ) ;
#10859=DIRECTION ( 'NONE',  ( -0.000000000000000000, 1.000000000000000000, -0.000000000000000000 ) ) ;
#10866=DIRECTION ( 'NONE',  ( 0.000000000000000000, 1.000000000000000000, 0.000000000000000000 ) ) ;
#10872=CLOSED_SHELL ( 'NONE', ( #7503, #19417, #19156, #8197, #18807, #384, #22572, #14915, #22018, #7032, #18992, #11887, #22585, #16071, #9332, #4836, #22699, #3771, #9541, #13204, #20309, #4025, #1486, #8510, #12361, #7223, #13896, #20583, #25286, #24751, #2606, #20998, #1435, #12760, #21847, #3854, #21362, #1605, #5839, #6286, #8903, #5375, #16448, #22360, #14147, #17505, #61, #12625, #8771, #7788, #7164, #20648, #8564, #18534, #25716, #1093, #11559 ) ) ;
#10873=ORIENTED_EDGE ( 'NONE', *, *, #14943, .F. ) ;
#10874=CIRCLE ( 'NONE', #7116, 6.000000000000000000 ) ;
#10883=CARTESIAN_POINT ( 'NONE',  ( 3.469446951953614189E-15, 39.50000000000000000, 8.999999999999992895 ) ) ;
#10900=EDGE_CURVE ( 'NONE', #4850, #12001, #19327, .T. ) ;
#10910=CARTESIAN_POINT ( 'NONE',  ( 1.878215178125003382, 29.37812499938548783, 5.746835883940462963 ) ) ;
#10914=AXIS2_PLACEMENT_3D ( 'NONE', #13166, #22971, #15373 ) ;
#10920=CARTESIAN_POINT ( 'NONE',  ( 0.000000000000000000, 25.92812499938548854, 13.33755215474603162 ) ) ;
#10924=CARTESIAN_POINT ( 'NONE',  ( -1.878215178124998275, 28.59062499938548640, 12.25316411605951927 ) ) ;
#10932=LINE ( 'NONE', #8711, #22195 ) ;
#10961=CARTESIAN_POINT ( 'NONE',  ( -3.756430356249997882, 28.62812499938548783, 8.999999999999992895 ) ) ;
#10963=AXIS2_PLACEMENT_3D ( 'NONE', #23893, #5709, #2185 ) ;
#10974=FACE_OUTER_BOUND ( 'NONE', #3584, .T. ) ;
#11004=AXIS2_PLACEMENT_3D ( 'NONE', #10883, #16926, #24894 ) ;
#11010=CARTESIAN_POINT ( 'NONE',  ( -3.999999999999994671, 29.70624999877097139, 11.30940107675849404 ) ) ;
#11015=ORIENTED_EDGE ( 'NONE', *, *, #16755, .T. ) ;
#11023=CIRCLE ( 'NONE', #18964, 6.000000000000000000 ) ;
#11037=CARTESIAN_POINT ( 'NONE',  ( -3.999999999999998224, 26.96874999877097068, 8.999999999999992895 ) ) ;
#11042=CARTESIAN_POINT ( 'NONE',  ( 1.878215178125003382, 29.67812499938549209, 12.25316411605952283 ) ) ;
#11043=EDGE_LOOP ( 'NONE', ( #12636, #22326, #25270, #5759 ) ) ;
#11051=CARTESIAN_POINT ( 'NONE',  ( 4.006172263299091013E-15, 25.25312499938549138, 4.662447845253954171 ) ) ;
#11053=DIRECTION ( 'NONE',  ( -0.000000000000000000, -1.000000000000000000, -0.000000000000000000 ) ) ;
#11054=CARTESIAN_POINT ( 'NONE',  ( -3.756430356249994773, 28.96562499938548640, 8.999999999999992895 ) ) ;
#11057=CARTESIAN_POINT ( 'NONE',  ( 4.000000000000003553, 25.45000000000000639, 8.999999999999992895 ) ) ;
#11081=ORIENTED_EDGE ( 'NONE', *, *, #10001, .T. ) ;
#11083=CARTESIAN_POINT ( 'NONE',  ( 1.878215178124999829, 26.97812499938549280, 12.25316411605952283 ) ) ;
#11098=LINE ( 'NONE', #23254, #17072 ) ;
#11104=CYLINDRICAL_SURFACE ( 'NONE', #17087, 0.5000000000000004441 ) ;
#11109=ORIENTED_EDGE ( 'NONE', *, *, #19844, .F. ) ;
#11111=VERTEX_POINT ( 'NONE', #22593 ) ;
#11133=VERTEX_POINT ( 'NONE', #10800 ) ;
#11136=CARTESIAN_POINT ( 'NONE',  ( 3.756430356250004987, 25.14062499938548356, 8.999999999999992895 ) ) ;
#11137=ORIENTED_EDGE ( 'NONE', *, *, #10309, .F. ) ;
#11154=ORIENTED_EDGE ( 'NONE', *, *, #7530, .F. ) ;
#11156=CARTESIAN_POINT ( 'NONE',  ( 0.000000000000000000, 26.63124999877097565, 13.61880215351699874 ) ) ;
#11164=CARTESIAN_POINT ( 'NONE',  ( 5.706339097770919189, 31.50000000000000000, 7.645898033750285983 ) ) ;
#11169=CARTESIAN_POINT ( 'NONE',  ( 3.756430356250003211, 29.19062499938548072, 8.999999999999992895 ) ) ;
#11170=CARTESIAN_POINT ( 'NONE',  ( 3.756430356250004099, 26.00312499938548783, 11.16877607737301403 ) ) ;
#11171=DIRECTION ( 'NONE',  ( 0.000000000000000000, 0.000000000000000000, 1.000000000000000000 ) ) ;
#11172=CARTESIAN_POINT ( 'NONE',  ( -1.999999999999996669, 25.15000000000000568, 5.535898384862237620 ) ) ;
#11173=CARTESIAN_POINT ( 'NONE',  ( 2.000000000000000000, 28.91874999877097707, 12.46410161513774817 ) ) ;
#11186=EDGE_CURVE ( 'NONE', #855, #25560, #11731, .T. ) ;
#11203=CARTESIAN_POINT ( 'NONE',  ( 3.756430356250004987, 26.60312499938548569, 8.999999999999992895 ) ) ;
#11225=CARTESIAN_POINT ( 'NONE',  ( -5.532151103383257329, 31.50000000000000000, 6.677220593914390712 ) ) ;
#11227=CARTESIAN_POINT ( 'NONE',  ( 3.756430356250004543, 29.71562499938548996, 11.16877607737301226 ) ) ;
#11236=ORIENTED_EDGE ( 'NONE', *, *, #13393, .T. ) ;
#11238=VERTEX_POINT ( 'NONE', #19428 ) ;
#11242=AXIS2_PLACEMENT_3D ( 'NONE', #14244, #639, #24163 ) ;
#11246=AXIS2_PLACEMENT_3D ( 'NONE', #6195, #463, #10363 ) ;
#11255=CARTESIAN_POINT ( 'NONE',  ( -2.000000000000000000, 25.30000000000001137, 12.46410161513774639 ) ) ;
#11274=EDGE_CURVE ( 'NONE', #6423, #17283, #24698, .T. ) ;
#11290=CARTESIAN_POINT ( 'NONE',  ( 4.000000000000002665, 26.70624999877097494, 11.30940107675849760 ) ) ;
#11297=EDGE_LOOP ( 'NONE', ( #5261, #15630, #23950, #9117 ) ) ;
#11305=CIRCLE ( 'NONE', #15458, 0.5000000000000004441 ) ;
#11308=CARTESIAN_POINT ( 'NONE',  ( 3.756430356250006319, 25.17812499938548854, 6.831223922626973533 ) ) ;
#11310=DIRECTION ( 'NONE',  ( 0.000000000000000000, 0.000000000000000000, -1.000000000000000000 ) ) ;
#11311=CARTESIAN_POINT ( 'NONE',  ( 3.756430356250004987, 29.64062499938548711, 8.999999999999992895 ) ) ;
#11314=CARTESIAN_POINT ( 'NONE',  ( 1.580380365229604700E-14, 27.58750000000000213, 12.99999999999999289 ) ) ;
#11340=DIRECTION ( 'NONE',  ( 0.000000000000000000, 0.000000000000000000, 1.000000000000000000 ) ) ;
#11342=CARTESIAN_POINT ( 'NONE',  ( -3.756430356250002323, 27.31562499938548783, 11.16877607737301226 ) ) ;
#11348=FILL_AREA_STYLE_COLOUR ( '', #14372 ) ;
#11366=CARTESIAN_POINT ( 'NONE',  ( 3.756430356250004543, 29.34062499938548640, 6.831223922626973533 ) ) ;
#11405=VERTEX_POINT ( 'NONE', #12228 ) ;
#11406=DIRECTION ( 'NONE',  ( 0.000000000000000000, 0.000000000000000000, 1.000000000000000000 ) ) ;
#11409=EDGE_LOOP ( 'NONE', ( #11727, #16376, #3555, #2375 ) ) ;
#11411=VECTOR ( 'NONE', #6825, 1000.000000000000000 ) ;
#11428=CARTESIAN_POINT ( 'NONE',  ( -3.999999999999996447, 28.28124999877097778, 6.690598923241487306 ) ) ;
#11439=ORIENTED_EDGE ( 'NONE', *, *, #12177, .F. ) ;
#11443=CARTESIAN_POINT ( 'NONE',  ( 3.756430356250002323, 27.42812499938548854, 6.831223922626973533 ) ) ;
#11445=CARTESIAN_POINT ( 'NONE',  ( 3.469446951953614189E-15, 25.00000000000000000, 8.999999999999992895 ) ) ;
#11446=CARTESIAN_POINT ( 'NONE',  ( -3.999999999999996447, 26.53750000000000497, 6.690598923241487306 ) ) ;
#11474=CARTESIAN_POINT ( 'NONE',  ( 2.003086131649545506E-15, 29.19062499938549138, 13.33755215474602984 ) ) ;
#11480=CARTESIAN_POINT ( 'NONE',  ( 4.000000000000007105, 28.60000000000000497, 8.999999999999992895 ) ) ;
#11495=CARTESIAN_POINT ( 'NONE',  ( 6.009258394948636914E-15, 29.41562499938548925, 4.662447845253954171 ) ) ;
#11501=EDGE_LOOP ( 'NONE', ( #21066, #19735, #14435, #18615 ) ) ;
#11505=CARTESIAN_POINT ( 'NONE',  ( -3.295251204612120066, 39.00010698140257404, 13.40411251903217327 ) ) ;
#11506=CARTESIAN_POINT ( 'NONE',  ( 3.756430356250003211, 25.59062499938548285, 8.999999999999992895 ) ) ;
#11510=( BOUNDED_CURVE ( )  B_SPLINE_CURVE ( 2, ( #19777, #5534, #7746, #19388, #21737 ),
 .UNSPECIFIED., .F., .F. ) 
 B_SPLINE_CURVE_WITH_KNOTS ( ( 3, 2, 3 ),
 ( 0.9749999999999999778, 0.9833333333333332815, 1.000000000000000000 ),
 .UNSPECIFIED. ) 
 CURVE ( )  GEOMETRIC_REPRESENTATION_ITEM ( )  RATIONAL_B_SPLINE_CURVE ( ( 0.9330127018922194093, 0.9330127018922194093, 1.000000000000000000, 0.8660254037844387076, 1.000000000000000000 ) ) 
 REPRESENTATION_ITEM ( '' )  );
#11532=ORIENTED_EDGE ( 'NONE', *, *, #6632, .T. ) ;
#11548=B_SPLINE_CURVE_WITH_KNOTS ( 'NONE', 3,
 ( #1902, #14055, #16149, #6194, #21901, #17592, #9987, #23604 ),
 .UNSPECIFIED., .F., .F.,
 ( 4, 2, 2, 4 ),
 ( 0.0009289288217882846459, 0.001160777380751506918, 0.001392625939714729408, 0.001856323057641173302 ),
 .UNSPECIFIED. ) ;
#11550=CARTESIAN_POINT ( 'NONE',  ( -1.999999999999998224, 27.04374999877097352, 12.46410161513774639 ) ) ;
#11557=CARTESIAN_POINT ( 'NONE',  ( 2.000000000000005329, 25.07500000000000284, 5.535898384862238508 ) ) ;
#11559=ADVANCED_FACE ( 'NONE', ( #6471 ), #1063, .T. ) ;
#11562=CARTESIAN_POINT ( 'NONE',  ( 0.000000000000000000, 28.62812499938549138, 13.33755215474603162 ) ) ;
#11565=CARTESIAN_POINT ( 'NONE',  ( 2.000000000000003553, 25.97500000000000497, 5.535898384862238508 ) ) ;
#11581=CARTESIAN_POINT ( 'NONE',  ( 1.878215178125003382, 25.32812499938548356, 5.746835883940462963 ) ) ;
#11584=( BOUNDED_CURVE ( )  B_SPLINE_CURVE ( 2, ( #18041, #24039, #13849, #251, #5865, #25872, #126, #14104, #12133 ),
 .UNSPECIFIED., .F., .F. ) 
 B_SPLINE_CURVE_WITH_KNOTS ( ( 3, 2, 2, 2, 3 ),
 ( 0.2750000000000000222, 0.2833333333333333259, 0.2999999999999999889, 0.3166666666666666519, 0.3250000000000000111 ),
 .UNSPECIFIED. ) 
 CURVE ( )  GEOMETRIC_REPRESENTATION_ITEM ( )  RATIONAL_B_SPLINE_CURVE ( ( 0.9330127018922194093, 0.9330127018922196314, 1.000000000000000000, 0.8660254037844387076, 1.000000000000000000, 0.8660254037844387076, 1.000000000000000000, 0.9330127018922191873, 0.9330127018922194093 ) ) 
 REPRESENTATION_ITEM ( '' )  );
#11590=CYLINDRICAL_SURFACE ( 'NONE', #2647, 4.000000000000000000 ) ;
#11591=CARTESIAN_POINT ( 'NONE',  ( -1.878215178124996498, 29.00312499938548783, 5.746835883940462963 ) ) ;
#11606=DIRECTION ( 'NONE',  ( -0.000000000000000000, -1.000000000000000000, -0.000000000000000000 ) ) ;
#11614=CARTESIAN_POINT ( 'NONE',  ( -5.357084559935323398, 38.69843056730299224, 6.772139184627471664 ) ) ;
#11617=ORIENTED_EDGE ( 'NONE', *, *, #24680, .T. ) ;
#11629=CARTESIAN_POINT ( 'NONE',  ( -1.071796769724485232, 27.83259618943233704, 4.999999999999992006 ) ) ;
#11636=DIRECTION ( 'NONE',  ( 0.000000000000000000, 0.000000000000000000, 1.000000000000000000 ) ) ;
#11666=CARTESIAN_POINT ( 'NONE',  ( -4.000000000000000000, 25.67500000000000426, 8.999999999999992895 ) ) ;
#11676=CARTESIAN_POINT ( 'NONE',  ( 1.487416814333745711E-14, 28.03750000000001208, 12.99999999999999289 ) ) ;
#11679=CARTESIAN_POINT ( 'NONE',  ( -3.756430356249996105, 25.44062499938548783, 6.831223922626973533 ) ) ;
#11684=CARTESIAN_POINT ( 'NONE',  ( -1.999999999999996669, 29.35000000000000853, 12.46410161513774639 ) ) ;
#11692=CARTESIAN_POINT ( 'NONE',  ( 3.077103717553398621, 38.94033362033496815, 4.369373194502302660 ) ) ;
#11694=CARTESIAN_POINT ( 'NONE',  ( -3.756430356249997882, 28.02812499938548996, 6.831223922626973533 ) ) ;
#11698=CARTESIAN_POINT ( 'NONE',  ( -3.999999999999998224, 26.12500000000001066, 8.999999999999992895 ) ) ;
#11700=DIRECTION ( 'NONE',  ( -0.000000000000000000, 1.000000000000000000, 0.000000000000000000 ) ) ;
#11708=EDGE_CURVE ( 'NONE', #8133, #17209, #11584, .T. ) ;
#11712=CARTESIAN_POINT ( 'NONE',  ( 4.000000000000002665, 27.23124999877097352, 6.690598923241489970 ) ) ;
#11713=VECTOR ( 'NONE', #14779, 1000.000000000000000 ) ;
#11716=ORIENTED_EDGE ( 'NONE', *, *, #22294, .F. ) ;
#11719=CARTESIAN_POINT ( 'NONE',  ( 1.878215178124999829, 25.62812499938549138, 12.25316411605952283 ) ) ;
#11727=ORIENTED_EDGE ( 'NONE', *, *, #18420, .F. ) ;
#11729=CARTESIAN_POINT ( 'NONE',  ( -1.878215178124999829, 29.15312499938549351, 12.25316411605951927 ) ) ;
#11731=CIRCLE ( 'NONE', #10069, 0.5000000000000004441 ) ;
#11740=CARTESIAN_POINT ( 'NONE',  ( 7.437084071668728555E-15, 26.63124999877097565, 12.99999999999999112 ) ) ;
#11745=( BOUNDED_CURVE ( )  B_SPLINE_CURVE ( 2, ( #20563, #2773, #14682, #10482, #6832, #8541, #12194, #2652, #22523 ),
 .UNSPECIFIED., .F., .F. ) 
 B_SPLINE_CURVE_WITH_KNOTS ( ( 3, 2, 2, 2, 3 ),
 ( 0.7249999999999999778, 0.7333333333333332815, 0.7500000000000000000, 0.7666666666666667185, 0.7750000000000000222 ),
 .UNSPECIFIED. ) 
 CURVE ( )  GEOMETRIC_REPRESENTATION_ITEM ( )  RATIONAL_B_SPLINE_CURVE ( ( 0.9330127018922194093, 0.9330127018922194093, 1.000000000000000000, 0.8660254037844387076, 1.000000000000000000, 0.8660254037844387076, 1.000000000000000000, 0.9330127018922194093, 0.9330127018922194093 ) ) 
 REPRESENTATION_ITEM ( '' )  );
#11750=CARTESIAN_POINT ( 'NONE',  ( 5.112995299272250684E-15, 26.01250000000000284, 4.999999999999992006 ) ) ;
#11752=VERTEX_POINT ( 'NONE', #12269 ) ;
#11753=CARTESIAN_POINT ( 'NONE',  ( -3.756430356249996549, 29.52812499938548996, 8.999999999999992895 ) ) ;
#11766=CARTESIAN_POINT ( 'NONE',  ( -1.071796769724483234, 28.01740381056767148, 12.99999999999999645 ) ) ;
#11786=CARTESIAN_POINT ( 'NONE',  ( 6.938893903907228378E-15, 29.50000000000000000, 2.999999999999992450 ) ) ;
#11791=VECTOR ( 'NONE', #15053, 1000.000000000000000 ) ;
#11814=CARTESIAN_POINT ( 'NONE',  ( -3.918623196469519065, 34.50000000000000000, 4.456389954662585140 ) ) ;
#11817=CARTESIAN_POINT ( 'NONE',  ( -4.000000000000000888, 29.25624999877096855, 11.30940107675849404 ) ) ;
#11831=CARTESIAN_POINT ( 'NONE',  ( 1.878215178125001605, 29.11562499938549209, 12.25316411605952283 ) ) ;
#11833=CARTESIAN_POINT ( 'NONE',  ( -4.000000000000000000, 27.47500000000000142, 8.999999999999992895 ) ) ;
#11851=EDGE_CURVE ( 'NONE', #22574, #2153, #7578, .T. ) ;
#11857=EDGE_CURVE ( 'NONE', #8259, #2175, #22734, .T. ) ;
#11858=CARTESIAN_POINT ( 'NONE',  ( 5.532151103383234236, 38.49999999999999289, 6.677220593914319657 ) ) ;
#11859=CARTESIAN_POINT ( 'NONE',  ( -1.878215178124998275, 29.60312499938548925, 12.25316411605951927 ) ) ;
#11874=CARTESIAN_POINT ( 'NONE',  ( 5.265192354984335132, 38.83322177420914301, 6.904532280874554395 ) ) ;
#11887=ADVANCED_FACE ( 'NONE', ( #4930 ), #12913, .T. ) ;
#11891=CARTESIAN_POINT ( 'NONE',  ( -3.756430356249998326, 28.10312499938548569, 11.16877607737301226 ) ) ;
#11895=( BOUNDED_CURVE ( )  B_SPLINE_CURVE ( 2, ( #19624, #24069, #17686, #10076, #16105, #25654, #18077, #5899, #9944 ),
 .UNSPECIFIED., .F., .F. ) 
 B_SPLINE_CURVE_WITH_KNOTS ( ( 3, 2, 2, 2, 3 ),
 ( 0.4250000000000000444, 0.4333333333333333481, 0.4500000000000000111, 0.4666666666666666741, 0.4750000000000000333 ),
 .UNSPECIFIED. ) 
 CURVE ( )  GEOMETRIC_REPRESENTATION_ITEM ( )  RATIONAL_B_SPLINE_CURVE ( ( 0.9330127018922194093, 0.9330127018922196314, 1.000000000000000000, 0.8660254037844387076, 1.000000000000000000, 0.8660254037844387076, 1.000000000000000000, 0.9330127018922191873, 0.9330127018922194093 ) ) 
 REPRESENTATION_ITEM ( '' )  );
#11907=CYLINDRICAL_SURFACE ( 'NONE', #556, 4.000000000000000000 ) ;
#11916=ORIENTED_EDGE ( 'NONE', *, *, #12700, .T. ) ;
#11935=CARTESIAN_POINT ( 'NONE',  ( 3.756430356250004543, 26.19062499938549138, 6.831223922626973533 ) ) ;
#11943=VERTEX_POINT ( 'NONE', #18799 ) ;
#11950=CARTESIAN_POINT ( 'NONE',  ( 6.009258394948636914E-15, 27.81250000000000711, 4.381197846482986158 ) ) ;
#11956=CARTESIAN_POINT ( 'NONE',  ( -3.526711513758413297, 38.89679573513893729, 4.645898033752330569 ) ) ;
#11966=CARTESIAN_POINT ( 'NONE',  ( 3.756430356250004099, 27.01562499938549067, 11.16877607737301403 ) ) ;
#11975=CARTESIAN_POINT ( 'NONE',  ( 6.009258394948636914E-15, 29.41562499938548925, 4.662447845253954171 ) ) ;
#11987=ORIENTED_EDGE ( 'NONE', *, *, #5950, .F. ) ;
#11993=CARTESIAN_POINT ( 'NONE',  ( 3.575950304376171562, 38.86679461760645182, 13.35281166003925613 ) ) ;
#12001=VERTEX_POINT ( 'NONE', #22458 ) ;
#12008=CARTESIAN_POINT ( 'NONE',  ( 1.878215178125003382, 27.46562499938548996, 5.746835883940462963 ) ) ;
#12018=DIRECTION ( 'NONE',  ( 0.000000000000000000, 0.000000000000000000, 1.000000000000000000 ) ) ;
#12025=DIRECTION ( 'NONE',  ( 1.000000000000000000, 0.000000000000000000, 0.000000000000000000 ) ) ;
#12045=CARTESIAN_POINT ( 'NONE',  ( 4.000000000000001776, 25.90000000000000568, 8.999999999999992895 ) ) ;
#12055=CARTESIAN_POINT ( 'NONE',  ( 3.918623196469491088, 31.50000000000000000, 13.54361004533742907 ) ) ;
#12056=ORIENTED_EDGE ( 'NONE', *, *, #389, .T. ) ;
#12059=CARTESIAN_POINT ( 'NONE',  ( 3.756430356250004543, 26.64062499938549067, 6.831223922626973533 ) ) ;
#12078=EDGE_CURVE ( 'NONE', #15395, #3609, #7775, .T. ) ;
#12081=CARTESIAN_POINT ( 'NONE',  ( -3.999999999999996447, 28.82500000000000284, 8.999999999999992895 ) ) ;
#12087=VECTOR ( 'NONE', #8667, 1000.000000000000000 ) ;
#12088=CARTESIAN_POINT ( 'NONE',  ( -3.688187414285967858, 38.77776551522837423, 4.624837864698400303 ) ) ;
#12100=CARTESIAN_POINT ( 'NONE',  ( -2.003086131649545506E-15, 26.49062499938548498, 13.33755215474603162 ) ) ;
#12109=CARTESIAN_POINT ( 'NONE',  ( -3.756430356250000546, 26.75312499938548783, 11.16877607737301226 ) ) ;
#12114=VECTOR ( 'NONE', #7260, 1000.000000000000114 ) ;
#12125=ORIENTED_EDGE ( 'NONE', *, *, #23050, .T. ) ;
#12130=CARTESIAN_POINT ( 'NONE',  ( 4.648177544792955347E-16, 29.33124999877097139, 12.99999999999999289 ) ) ;
#12133=CARTESIAN_POINT ( 'NONE',  ( -4.648177544792955347E-16, 26.85624999877096997, 4.999999999999991118 ) ) ;
#12137=VERTEX_POINT ( 'NONE', #1187 ) ;
#12141=EDGE_CURVE ( 'NONE', #3500, #13892, #17220, .T. ) ;
#12146=CARTESIAN_POINT ( 'NONE',  ( -1.878215178124994722, 25.40312499938548996, 5.746835883940462963 ) ) ;
#12148=VECTOR ( 'NONE', #6741, 1000.000000000000000 ) ;
#12149=CARTESIAN_POINT ( 'NONE',  ( 3.756430356250004543, 26.00312499938548783, 11.16877607737301226 ) ) ;
#12159=CARTESIAN_POINT ( 'NONE',  ( -5.706339097770935176, 29.50000000000000000, 7.145898033750358813 ) ) ;
#12164=CARTESIAN_POINT ( 'NONE',  ( 4.000000000000005329, 28.05624999877096926, 11.30940107675849760 ) ) ;
#12171=EDGE_CURVE ( 'NONE', #14315, #1503, #7338, .T. ) ;
#12172=ORIENTED_EDGE ( 'NONE', *, *, #15359, .F. ) ;
#12177=EDGE_CURVE ( 'NONE', #7296, #20975, #9281, .T. ) ;
#12194=CARTESIAN_POINT ( 'NONE',  ( -1.999999999999998224, 28.84374999877097423, 12.46410161513774639 ) ) ;
#12202=CARTESIAN_POINT ( 'NONE',  ( -3.756430356249996105, 26.34062499938548285, 6.831223922626973533 ) ) ;
#12203=VECTOR ( 'NONE', #21426, 1000.000000000000000 ) ;
#12207=VERTEX_POINT ( 'NONE', #25258 ) ;
#12208=DIRECTION ( 'NONE',  ( 3.552713678800501718E-15, 0.000000000000000000, 1.000000000000000000 ) ) ;
#12213=ORIENTED_EDGE ( 'NONE', *, *, #15240, .T. ) ;
#12220=CARTESIAN_POINT ( 'NONE',  ( 4.000000000000002665, 29.01250000000000284, 11.30940107675849760 ) ) ;
#12228=CARTESIAN_POINT ( 'NONE',  ( 3.110308778861319734, 31.50000000000000000, 3.869115154270335477 ) ) ;
#12235=CARTESIAN_POINT ( 'NONE',  ( -3.756430356249997882, 27.24062499938548854, 6.831223922626973533 ) ) ;
#12239=CYLINDRICAL_SURFACE ( 'NONE', #1287, 0.5000000000000004441 ) ;
#12244=CARTESIAN_POINT ( 'NONE',  ( -3.756430356249996105, 29.00312499938548427, 11.16877607737301226 ) ) ;
#12257=CARTESIAN_POINT ( 'NONE',  ( -1.071796769724485232, 26.42634618820330772, 4.999999999999992006 ) ) ;
#12266=CARTESIAN_POINT ( 'NONE',  ( 4.648177544792954952E-15, 25.73124999877097707, 12.99999999999999289 ) ) ;
#12269=CARTESIAN_POINT ( 'NONE',  ( 0.4995657836784155315, 31.50000000000000000, 3.020833333333325044 ) ) ;
#12276=VERTEX_POINT ( 'NONE', #7598 ) ;
#12281=CARTESIAN_POINT ( 'NONE',  ( -3.756430356249996105, 25.96562499938548996, 11.16877607737301226 ) ) ;
#12298=CARTESIAN_POINT ( 'NONE',  ( 1.533898589781675205E-14, 27.98124999877097352, 12.99999999999999289 ) ) ;
#12331=CARTESIAN_POINT ( 'NONE',  ( 2.003086131649545506E-15, 26.94062499938549138, 13.33755215474602984 ) ) ;
#12352=CARTESIAN_POINT ( 'NONE',  ( 2.006336132164985451E-12, 39.00000000001113420, 3.500000000010202061 ) ) ;
#12354=CARTESIAN_POINT ( 'NONE',  ( -3.999999999999998224, 25.61874999877097281, 8.999999999999992895 ) ) ;
#12361=ADVANCED_FACE ( 'NONE', ( #4178 ), #19991, .T. ) ;
#12362=CARTESIAN_POINT ( 'NONE',  ( 1.878215178125001605, 26.52812499938548640, 12.25316411605952283 ) ) ;
#12364=VERTEX_POINT ( 'NONE', #17795 ) ;
#12365=FACE_OUTER_BOUND ( 'NONE', #16654, .T. ) ;
#12367=CARTESIAN_POINT ( 'NONE',  ( 3.688104818422799358, 38.77776441442690469, 4.624767765505003680 ) ) ;
#12372=CARTESIAN_POINT ( 'NONE',  ( 0.000000000000000000, 27.72812499938548925, 13.33755215474602984 ) ) ;
#12387=ORIENTED_EDGE ( 'NONE', *, *, #5782, .T. ) ;
#12392=DIRECTION ( 'NONE',  ( -0.000000000000000000, -1.000000000000000000, -0.000000000000000000 ) ) ;
#12403=CARTESIAN_POINT ( 'NONE',  ( 4.006172263299091013E-15, 25.36562499938549564, 4.662447845253954171 ) ) ;
#12412=LINE ( 'NONE', #10579, #17054 ) ;
#12415=CARTESIAN_POINT ( 'NONE',  ( -3.999999999999999112, 27.51250000000000995, 11.30940107675849404 ) ) ;
#12423=( BOUNDED_CURVE ( )  B_SPLINE_CURVE ( 2, ( #12298, #155, #13745, #12164, #5896, #10073, #18074, #14133, #8125 ),
 .UNSPECIFIED., .F., .T. ) 
 B_SPLINE_CURVE_WITH_KNOTS ( ( 3, 2, 2, 2, 3 ),
 ( 0.5750000000000000666, 0.5833333333333333703, 0.5999999999999999778, 0.6166666666666666963, 0.6250000000000000000 ),
 .UNSPECIFIED. ) 
 CURVE ( )  GEOMETRIC_REPRESENTATION_ITEM ( )  RATIONAL_B_SPLINE_CURVE ( ( 0.9330127018922194093, 0.9330127018922198534, 1.000000000000000000, 0.8660254037844387076, 1.000000000000000000, 0.8660254037844387076, 1.000000000000000000, 0.9330127018922194093, 0.9330127018922194093 ) ) 
 REPRESENTATION_ITEM ( '' )  );
#12427=ORIENTED_EDGE ( 'NONE', *, *, #8266, .F. ) ;
#12428=ORIENTED_EDGE ( 'NONE', *, *, #19709, .F. ) ;
#12431=( BOUNDED_CURVE ( )  B_SPLINE_CURVE ( 2, ( #4050, #7602, #19997, #23675, #15831, #21470, #7726, #1969, #5892 ),
 .UNSPECIFIED., .F., .F. ) 
 B_SPLINE_CURVE_WITH_KNOTS ( ( 3, 2, 2, 2, 3 ),
 ( 0.5750000000000000666, 0.5833333333333333703, 0.5999999999999999778, 0.6166666666666666963, 0.6250000000000000000 ),
 .UNSPECIFIED. ) 
 CURVE ( )  GEOMETRIC_REPRESENTATION_ITEM ( )  RATIONAL_B_SPLINE_CURVE ( ( 0.9330127018922194093, 0.9330127018922198534, 1.000000000000000000, 0.8660254037844387076, 1.000000000000000000, 0.8660254037844387076, 1.000000000000000000, 0.9330127018922194093, 0.9330127018922194093 ) ) 
 REPRESENTATION_ITEM ( '' )  );
#12451=CARTESIAN_POINT ( 'NONE',  ( -1.878215178124998275, 28.25312499938548783, 12.25316411605951927 ) ) ;
#12455=CARTESIAN_POINT ( 'NONE',  ( -1.999999999999998224, 28.45000000000000639, 12.46410161513774639 ) ) ;
#12464=LINE ( 'NONE', #16540, #1358 ) ;
#12466=DIRECTION ( 'NONE',  ( 0.000000000000000000, -0.000000000000000000, 1.000000000000000000 ) ) ;
#12473=CARTESIAN_POINT ( 'NONE',  ( -0.07793552093707546702, 39.00000000000049027, 3.500000000000446754 ) ) ;
#12474=CARTESIAN_POINT ( 'NONE',  ( 4.000000000000005329, 25.43124999877097281, 6.690598923241489970 ) ) ;
#12484=CARTESIAN_POINT ( 'NONE',  ( -1.878215178124999829, 28.70312499938548711, 12.25316411605951927 ) ) ;
#12493=CARTESIAN_POINT ( 'NONE',  ( 1.878215178125003382, 27.46562499938548996, 5.746835883940462963 ) ) ;
#12496=CIRCLE ( 'NONE', #6654, 4.000000000000000000 ) ;
#12503=EDGE_CURVE ( 'NONE', #24856, #25109, #8551, .T. ) ;
#12507=CIRCLE ( 'NONE', #15863, 0.5000000000000004441 ) ;
#12528=EDGE_LOOP ( 'NONE', ( #3585, #9023, #24203, #17337, #8581, #24344, #9411, #20154, #14148, #17552, #10645, #19550, #8253, #13748, #25029, #3944, #17424, #23243, #22075, #11987, #14527, #11716, #7415, #18315, #13751 ) ) ;
#12554=ORIENTED_EDGE ( 'NONE', *, *, #4797, .F. ) ;
#12555=DIRECTION ( 'NONE',  ( -0.000000000000000000, -1.000000000000000000, -0.000000000000000000 ) ) ;
#12584=( BOUNDED_CURVE ( )  B_SPLINE_CURVE ( 2, ( #21987, #20765, #14496, #18673, #759 ),
 .UNSPECIFIED., .F., .T. ) 
 B_SPLINE_CURVE_WITH_KNOTS ( ( 3, 2, 3 ),
 ( 0.9749999999999999778, 0.9833333333333332815, 1.000000000000000000 ),
 .UNSPECIFIED. ) 
 CURVE ( )  GEOMETRIC_REPRESENTATION_ITEM ( )  RATIONAL_B_SPLINE_CURVE ( ( 0.9330127018922194093, 0.9330127018922194093, 1.000000000000000000, 0.8660254037844387076, 1.000000000000000000 ) ) 
 REPRESENTATION_ITEM ( '' )  );
#12585=CARTESIAN_POINT ( 'NONE',  ( 0.000000000000000000, 29.78124999877097423, 12.99999999999999289 ) ) ;
#12591=CARTESIAN_POINT ( 'NONE',  ( -3.756430356250000546, 28.21562499938548640, 11.16877607737301226 ) ) ;
#12602=AXIS2_PLACEMENT_3D ( 'NONE', #2290, #21774, #22160 ) ;
#12609=CARTESIAN_POINT ( 'NONE',  ( 3.469446951953614189E-15, 35.50000000000000711, 4.999999999999992006 ) ) ;
#12610=CARTESIAN_POINT ( 'NONE',  ( -1.071796769724489895, 26.66740381056767006, 12.99999999999999289 ) ) ;
#12612=AXIS2_PLACEMENT_3D ( 'NONE', #16349, #24318, #20743 ) ;
#12621=CARTESIAN_POINT ( 'NONE',  ( -3.999999999999996447, 25.58124999877097494, 6.690598923241487306 ) ) ;
#12625=ADVANCED_FACE ( 'NONE', ( #17632 ), #3237, .F. ) ;
#12636=ORIENTED_EDGE ( 'NONE', *, *, #6855, .F. ) ;
#12638=CARTESIAN_POINT ( 'NONE',  ( 3.756430356250003211, 28.74062499938548498, 8.999999999999992895 ) ) ;
#12642=CARTESIAN_POINT ( 'NONE',  ( 3.756430356250002323, 27.42812499938548498, 6.831223922626973533 ) ) ;
#12657=LINE ( 'NONE', #8991, #14986 ) ;
#12667=ORIENTED_EDGE ( 'NONE', *, *, #23305, .F. ) ;
#12682=CARTESIAN_POINT ( 'NONE',  ( -3.041313392017702455, 38.65031218604096352, 4.002974454653567271 ) ) ;
#12696=ORIENTED_EDGE ( 'NONE', *, *, #6858, .F. ) ;
#12700=EDGE_CURVE ( 'NONE', #2753, #25495, #23249, .T. ) ;
#12711=DIRECTION ( 'NONE',  ( 0.000000000000000000, 0.000000000000000000, -1.000000000000000000 ) ) ;
#12714=DIRECTION ( 'NONE',  ( 0.000000000000000000, 0.000000000000000000, -1.000000000000000000 ) ) ;
#12728=CARTESIAN_POINT ( 'NONE',  ( -3.756430356249998326, 29.04062499938548569, 6.831223922626973533 ) ) ;
#12734=ORIENTED_EDGE ( 'NONE', *, *, #14533, .F. ) ;
#12743=DIRECTION ( 'NONE',  ( -0.000000000000000000, -1.000000000000000000, -0.000000000000000000 ) ) ;
#12747=CARTESIAN_POINT ( 'NONE',  ( 3.469446951953614189E-15, 31.50000000000000000, 8.999999999999992895 ) ) ;
#12758=CARTESIAN_POINT ( 'NONE',  ( -3.756430356249994773, 29.07812499938548711, 8.999999999999992895 ) ) ;
#12760=ADVANCED_FACE ( 'NONE', ( #6104 ), #7940, .T. ) ;
#12763=EDGE_CURVE ( 'NONE', #7410, #11752, #4272, .T. ) ;
#12768=CARTESIAN_POINT ( 'NONE',  ( 1.878215178125006934, 26.56562499938548783, 5.746835883940462963 ) ) ;
#12771=CARTESIAN_POINT ( 'NONE',  ( 4.006172263299091013E-15, 25.33750000000000924, 13.61880215351699874 ) ) ;
#12773=CARTESIAN_POINT ( 'NONE',  ( 4.648177544792955347E-16, 28.93750000000000355, 12.99999999999999289 ) ) ;
#12799=CARTESIAN_POINT ( 'NONE',  ( 1.878215178125001605, 27.87812499938548783, 12.25316411605952283 ) ) ;
#12800=EDGE_CURVE ( 'NONE', #3609, #4893, #15788, .T. ) ;
#12807=UNCERTAINTY_MEASURE_WITH_UNIT (LENGTH_MEASURE( 1.000000000000000082E-05 ), #8621, 'distance_accuracy_value', 'NONE');
#12871=CARTESIAN_POINT ( 'NONE',  ( -1.999999999999996669, 26.59374999877097423, 12.46410161513774639 ) ) ;
#12889=CARTESIAN_POINT ( 'NONE',  ( 4.000000000000001776, 25.00000000000000000, 8.999999999999992895 ) ) ;
#12894=CARTESIAN_POINT ( 'NONE',  ( 1.071796769724495446, 25.54240381056767362, 4.999999999999992895 ) ) ;
#12895=VECTOR ( 'NONE', #1816, 1000.000000000000000 ) ;
#12913=CYLINDRICAL_SURFACE ( 'NONE', #1327, 4.000000000000000000 ) ;
#12926=CARTESIAN_POINT ( 'NONE',  ( -3.756430356249997882, 27.72812499938548569, 8.999999999999992895 ) ) ;
#12927=AXIS2_PLACEMENT_3D ( 'NONE', #6165, #2126, #9837 ) ;
#12936=CARTESIAN_POINT ( 'NONE',  ( -5.532151103383211144, 34.50000000000000000, 11.32277940608570255 ) ) ;
#12973=CARTESIAN_POINT ( 'NONE',  ( -4.648177544792955347E-16, 27.08124999877097139, 12.99999999999999289 ) ) ;
#12985=CIRCLE ( 'NONE', #16326, 0.5000000000000000000 ) ;
#13009=CARTESIAN_POINT ( 'NONE',  ( 4.000000000000002665, 27.68124999877097281, 6.690598923241489970 ) ) ;
#13019=ORIENTED_EDGE ( 'NONE', *, *, #21668, .T. ) ;
#13022=VECTOR ( 'NONE', #11606, 1000.000000000000000 ) ;
#13024=ORIENTED_EDGE ( 'NONE', *, *, #12141, .T. ) ;
#13027=CARTESIAN_POINT ( 'NONE',  ( -3.756430356249997882, 29.41562499938548569, 8.999999999999992895 ) ) ;
#13028=CARTESIAN_POINT ( 'NONE',  ( 4.006172263299091013E-15, 25.47812499938548925, 13.33755215474603162 ) ) ;
#13032=CARTESIAN_POINT ( 'NONE',  ( -3.756430356249998326, 29.45312499938549422, 11.16877607737301226 ) ) ;
#13045=CARTESIAN_POINT ( 'NONE',  ( 4.648177544792955347E-16, 28.48750000000000071, 12.99999999999999289 ) ) ;
#13062=VERTEX_POINT ( 'NONE', #18653 ) ;
#13064=CARTESIAN_POINT ( 'NONE',  ( 1.878215178125003382, 26.67812499938548854, 5.746835883940462963 ) ) ;
#13072=CARTESIAN_POINT ( 'NONE',  ( -7.901901826148023498E-15, 28.71250000000000568, 4.999999999999992006 ) ) ;
#13077=DIRECTION ( 'NONE',  ( -0.000000000000000000, -1.000000000000000000, -0.000000000000000000 ) ) ;
#13085=CARTESIAN_POINT ( 'NONE',  ( -3.526711513754876570, 29.50000000000000000, 4.145898033750337497 ) ) ;
#13087=DIRECTION ( 'NONE',  ( 0.000000000000000000, 1.000000000000000000, 0.000000000000000000 ) ) ;
#13112=CARTESIAN_POINT ( 'NONE',  ( -5.752022074721577560, 38.59074972337092646, 7.645898033750358813 ) ) ;
#13118=ORIENTED_EDGE ( 'NONE', *, *, #2634, .F. ) ;
#13120=CYLINDRICAL_SURFACE ( 'NONE', #5843, 6.000000000000000888 ) ;
#13124=VERTEX_POINT ( 'NONE', #11314 ) ;
#13146=CARTESIAN_POINT ( 'NONE',  ( -3.999999999999998224, 28.76874999877097139, 8.999999999999992895 ) ) ;
#13155=ORIENTED_EDGE ( 'NONE', *, *, #4335, .F. ) ;
#13158=CARTESIAN_POINT ( 'NONE',  ( 1.878215178125001605, 25.96562499938548996, 12.25316411605952283 ) ) ;
#13160=CARTESIAN_POINT ( 'NONE',  ( 2.000000000000005329, 25.52500000000000568, 5.535898384862238508 ) ) ;
#13166=CARTESIAN_POINT ( 'NONE',  ( 3.469446951953614189E-15, 39.50000000000000000, 8.999999999999992895 ) ) ;
#13168=DIRECTION ( 'NONE',  ( 0.8660254037844395958, 0.4999999999999982792, 0.000000000000000000 ) ) ;
#13172=DIRECTION ( 'NONE',  ( 0.000000000000000000, 1.000000000000000000, 0.000000000000000000 ) ) ;
#13189=CARTESIAN_POINT ( 'NONE',  ( 0.000000000000000000, 27.84062499938548996, 13.33755215474602984 ) ) ;
#13192=SURFACE_SIDE_STYLE ('',( #9648 ) ) ;
#13193=DIRECTION ( 'NONE',  ( -0.000000000000000000, 1.000000000000000000, -0.000000000000000000 ) ) ;
#13204=ADVANCED_FACE ( 'NONE', ( #17595 ), #21015, .T. ) ;
#13223=DIRECTION ( 'NONE',  ( 1.000000000000000000, 0.000000000000000000, 0.000000000000000000 ) ) ;
#13244=ORIENTED_EDGE ( 'NONE', *, *, #17901, .F. ) ;
#13251=CARTESIAN_POINT ( 'NONE',  ( 5.112995299272250684E-15, 25.56250000000000711, 4.999999999999992006 ) ) ;
#13259=CARTESIAN_POINT ( 'NONE',  ( -1.999999999999996669, 27.94374999877097565, 12.46410161513774639 ) ) ;
#13268=( BOUNDED_CURVE ( )  B_SPLINE_CURVE ( 2, ( #13280, #8982, #11173, #24925, #25673, #22966, #21254, #1753, #9723 ),
 .UNSPECIFIED., .F., .F. ) 
 B_SPLINE_CURVE_WITH_KNOTS ( ( 3, 2, 2, 2, 3 ),
 ( 0.7750000000000000222, 0.7833333333333333259, 0.8000000000000000444, 0.8166666666666666519, 0.8250000000000000666 ),
 .UNSPECIFIED. ) 
 CURVE ( )  GEOMETRIC_REPRESENTATION_ITEM ( )  RATIONAL_B_SPLINE_CURVE ( ( 0.9330127018922194093, 0.9330127018922194093, 1.000000000000000000, 0.8660254037844387076, 1.000000000000000000, 0.8660254037844387076, 1.000000000000000000, 0.9330127018922189652, 0.9330127018922194093 ) ) 
 REPRESENTATION_ITEM ( '' )  );
#13276=( BOUNDED_CURVE ( )  B_SPLINE_CURVE ( 2, ( #21815, #12257, #5985, #10161, #236, #6108, #10402, #22198, #14092 ),
 .UNSPECIFIED., .F., .F. ) 
 B_SPLINE_CURVE_WITH_KNOTS ( ( 3, 2, 2, 2, 3 ),
 ( 0.2250000000000000056, 0.2333333333333333370, 0.2500000000000000000, 0.2666666666666666630, 0.2750000000000000222 ),
 .UNSPECIFIED. ) 
 CURVE ( )  GEOMETRIC_REPRESENTATION_ITEM ( )  RATIONAL_B_SPLINE_CURVE ( ( 0.9330127018922194093, 0.9330127018922194093, 1.000000000000000000, 0.8660254037844387076, 1.000000000000000000, 0.8660254037844387076, 1.000000000000000000, 0.9330127018922191873, 0.9330127018922194093 ) ) 
 REPRESENTATION_ITEM ( '' )  );
#13277=CARTESIAN_POINT ( 'NONE',  ( -3.756430356249997882, 26.26562499938548711, 8.999999999999992895 ) ) ;
#13279=CARTESIAN_POINT ( 'NONE',  ( 1.878215178125005158, 28.81562499938548783, 5.746835883940462963 ) ) ;
#13280=CARTESIAN_POINT ( 'NONE',  ( 1.394453263437886604E-15, 28.88124999877097210, 12.99999999999999289 ) ) ;
#13307=ORIENTED_EDGE ( 'NONE', *, *, #14470, .T. ) ;
#13310=CARTESIAN_POINT ( 'NONE',  ( 3.756430356250004543, 26.64062499938549067, 6.831223922626973533 ) ) ;
#13344=ORIENTED_EDGE ( 'NONE', *, *, #12078, .F. ) ;
#13348=CARTESIAN_POINT ( 'NONE',  ( -1.999999999999998224, 28.00000000000000711, 12.46410161513774639 ) ) ;
#13353=CARTESIAN_POINT ( 'NONE',  ( 0.000000000000000000, 0.000000000000000000, 0.000000000000000000 ) ) ;
#13354=( BOUNDED_CURVE ( )  B_SPLINE_CURVE ( 2, ( #3403, #11629, #5361, #9681, #1571, #25252, #13348, #11766, #25501 ),
 .UNSPECIFIED., .F., .F. ) 
 B_SPLINE_CURVE_WITH_KNOTS ( ( 3, 2, 2, 2, 3 ),
 ( 0.6250000000000000000, 0.6333333333333333037, 0.6500000000000000222, 0.6666666666666666297, 0.6750000000000000444 ),
 .UNSPECIFIED. ) 
 CURVE ( )  GEOMETRIC_REPRESENTATION_ITEM ( )  RATIONAL_B_SPLINE_CURVE ( ( 0.9330127018922194093, 0.9330127018922194093, 1.000000000000000000, 0.8660254037844387076, 1.000000000000000000, 0.8660254037844387076, 1.000000000000000000, 0.9330127018922189652, 0.9330127018922194093 ) ) 
 REPRESENTATION_ITEM ( '' )  );
#13367=DIRECTION ( 'NONE',  ( 0.000000000000000000, 0.000000000000000000, -1.000000000000000000 ) ) ;
#13374=FACE_OUTER_BOUND ( 'NONE', #6449, .T. ) ;
#13386=CARTESIAN_POINT ( 'NONE',  ( -1.999999999999993117, 25.60000000000000497, 5.535898384862237620 ) ) ;
#13389=VECTOR ( 'NONE', #24818, 1000.000000000000000 ) ;
#13393=EDGE_CURVE ( 'NONE', #4850, #3500, #18718, .T. ) ;
#13398=CARTESIAN_POINT ( 'NONE',  ( -3.999999999999996447, 27.38124999877097210, 6.690598923241487306 ) ) ;
#13400=VERTEX_POINT ( 'NONE', #7080 ) ;
#13415=CARTESIAN_POINT ( 'NONE',  ( 3.756430356250002323, 27.35312499938548569, 11.16877607737301403 ) ) ;
#13417=B_SPLINE_CURVE_WITH_KNOTS ( 'NONE', 3,
 ( #6730, #24123, #22560, #2552, #605, #2683, #18374, #2805, #475, #4257, #4644, #8444, #16674, #16160, #849, #4502 ),
 .UNSPECIFIED., .F., .F.,
 ( 4, 2, 2, 2, 2, 2, 2, 4 ),
 ( 2.789812634830972505E-07, 0.0002322844908106880453, 0.0004642900003578929839, 0.0006962955099050979497, 0.0009283010194523028070, 0.001160306528999507664, 0.001392312038546712847, 0.001856323057641127115 ),
 .UNSPECIFIED. ) ;
#13418=DIRECTION ( 'NONE',  ( 0.000000000000000000, 1.000000000000000000, 0.000000000000000000 ) ) ;
#13419=CARTESIAN_POINT ( 'NONE',  ( -3.999999999999996447, 27.06250000000000711, 11.30940107675849404 ) ) ;
#13420=B_SPLINE_CURVE_WITH_KNOTS ( 'NONE', 3,
 ( #9785, #23909, #6377, #19962, #17765, #25734, #10034, #2066, #7817, #15798, #18032, #118, #13841, #1941, #4674, #2831 ),
 .UNSPECIFIED., .F., .F.,
 ( 4, 2, 2, 2, 2, 2, 2, 4 ),
 ( 2.789812634831446314E-07, 0.0002322844908106895361, 0.0004642900003578959655, 0.0006962955099051023949, 0.0009283010194523087701, 0.001160306528999515037, 0.001392312038546721521, 0.001856323057641130585 ),
 .UNSPECIFIED. ) ;
#13428=LINE ( 'NONE', #7522, #5370 ) ;
#13431=DIRECTION ( 'NONE',  ( 0.000000000000000000, 0.000000000000000000, 1.000000000000000000 ) ) ;
#13437=CARTESIAN_POINT ( 'NONE',  ( 4.000000000000002665, 25.80624999877096926, 11.30940107675849760 ) ) ;
#13442=CARTESIAN_POINT ( 'NONE',  ( 3.756430356250002323, 25.66562499938548925, 11.16877607737301403 ) ) ;
#13453=CARTESIAN_POINT ( 'NONE',  ( 4.006172263299091013E-15, 25.25312499938549138, 4.662447845253954171 ) ) ;
#13467=VERTEX_POINT ( 'NONE', #6830 ) ;
#13472=CIRCLE ( 'NONE', #2189, 6.000000000000000000 ) ;
#13476=ORIENTED_EDGE ( 'NONE', *, *, #16826, .F. ) ;
#13477=CARTESIAN_POINT ( 'NONE',  ( 1.878215178125003382, 29.37812499938548783, 5.746835883940462963 ) ) ;
#13485=ORIENTED_EDGE ( 'NONE', *, *, #24866, .T. ) ;
#13487=CARTESIAN_POINT ( 'NONE',  ( -3.079592406726821441, 38.55544002051693298, 14.08467396235847069 ) ) ;
#13503=FACE_OUTER_BOUND ( 'NONE', #11501, .T. ) ;
#13514=EDGE_LOOP ( 'NONE', ( #8002, #4874, #15692, #25219 ) ) ;
#13527=CARTESIAN_POINT ( 'NONE',  ( 4.000000000000005329, 28.18750000000000000, 6.690598923241489970 ) ) ;
#13531=CARTESIAN_POINT ( 'NONE',  ( 2.000000000000005329, 26.81874999877097210, 5.535898384862238508 ) ) ;
#13543=CARTESIAN_POINT ( 'NONE',  ( 3.162936011776061651, 38.99381541083456426, 4.492646367981153688 ) ) ;
#13545=CARTESIAN_POINT ( 'NONE',  ( -3.756430356249996549, 28.47812499938548569, 6.831223922626973533 ) ) ;
#13548=CARTESIAN_POINT ( 'NONE',  ( 0.000000000000000000, 27.13750000000000639, 13.61880215351699874 ) ) ;
#13574=CARTESIAN_POINT ( 'NONE',  ( 4.006172263299091013E-15, 25.47812499938548925, 13.33755215474602984 ) ) ;
#13579=CARTESIAN_POINT ( 'NONE',  ( 1.071796769724490561, 28.69240381056766864, 4.999999999999988454 ) ) ;
#13592=CARTESIAN_POINT ( 'NONE',  ( 3.509827456141323410, 38.91143067427094593, 13.34938134445224911 ) ) ;
#13626=ORIENTED_EDGE ( 'NONE', *, *, #4873, .F. ) ;
#13644=CARTESIAN_POINT ( 'NONE',  ( 3.469446951953614189E-15, 39.50000000000000000, 8.999999999999992895 ) ) ;
#13646=CARTESIAN_POINT ( 'NONE',  ( 4.000000000000000888, 28.11250000000000071, 11.30940107675849760 ) ) ;
#13649=CARTESIAN_POINT ( 'NONE',  ( 4.000000000000002665, 29.40624999877096357, 11.30940107675849760 ) ) ;
#13654=ORIENTED_EDGE ( 'NONE', *, *, #17402, .T. ) ;
#13660=CARTESIAN_POINT ( 'NONE',  ( 2.003086131649545506E-15, 29.07812499938549067, 13.33755215474603162 ) ) ;
#13662=CARTESIAN_POINT ( 'NONE',  ( -3.999999999999996447, 27.92500000000000426, 8.999999999999992895 ) ) ;
#13674=CARTESIAN_POINT ( 'NONE',  ( 4.000000000000000888, 27.15624999877097423, 11.30940107675849760 ) ) ;
#13680=CARTESIAN_POINT ( 'NONE',  ( 1.878215178125005158, 25.77812499938548996, 5.746835883940462963 ) ) ;
#13683=DIRECTION ( 'NONE',  ( 0.000000000000000000, 0.000000000000000000, 1.000000000000000000 ) ) ;
#13689=CARTESIAN_POINT ( 'NONE',  ( 3.756430356250004543, 26.07812499938549422, 6.831223922626973533 ) ) ;
#13695=SHAPE_REPRESENTATION_RELATIONSHIP ( 'NONE' , 'NONE' ,  #22515, #4445 ) ;
#13712=CARTESIAN_POINT ( 'NONE',  ( -5.532151103383257329, 38.49999999999999289, 6.677220593914388935 ) ) ;
#13720=CARTESIAN_POINT ( 'NONE',  ( -3.369773278825879181, 38.97868814324865383, 13.37417080150618354 ) ) ;
#13728=B_SPLINE_CURVE_WITH_KNOTS ( 'NONE', 3,
 ( #21554, #3381, #5343, #5607 ),
 .UNSPECIFIED., .F., .F.,
 ( 4, 4 ),
 ( 0.001666568017356004870, 0.001856323057641126682 ),
 .UNSPECIFIED. ) ;
#13732=LINE ( 'NONE', #23551, #10857 ) ;
#13745=CARTESIAN_POINT ( 'NONE',  ( 2.000000000000000000, 28.01874999877097139, 12.46410161513774817 ) ) ;
#13748=ORIENTED_EDGE ( 'NONE', *, *, #7657, .F. ) ;
#13751=ORIENTED_EDGE ( 'NONE', *, *, #20794, .T. ) ;
#13764=CARTESIAN_POINT ( 'NONE',  ( -1.999999999999993117, 27.34374999877097068, 5.535898384862237620 ) ) ;
#13766=DIRECTION ( 'NONE',  ( -0.000000000000000000, -1.000000000000000000, -0.000000000000000000 ) ) ;
#13779=CARTESIAN_POINT ( 'NONE',  ( 4.000000000000002665, 29.03124999877097423, 6.690598923241489970 ) ) ;
#13791=CARTESIAN_POINT ( 'NONE',  ( 0.4860084296119324132, 38.61007524145222192, 14.86986133562586865 ) ) ;
#13793=CARTESIAN_POINT ( 'NONE',  ( 3.756430356250003211, 27.39062499938548711, 8.999999999999992895 ) ) ;
#13797=CARTESIAN_POINT ( 'NONE',  ( -1.999999999999994893, 26.05000000000000426, 5.535898384862237620 ) ) ;
#13816=CARTESIAN_POINT ( 'NONE',  ( 3.756430356250003211, 26.15312499938548996, 8.999999999999992895 ) ) ;
#13827=CARTESIAN_POINT ( 'NONE',  ( -3.756430356249998326, 29.04062499938548569, 6.831223922626973533 ) ) ;
#13833=CARTESIAN_POINT ( 'NONE',  ( 6.938893903907228378E-15, 31.50000000000000000, 2.999999999999992450 ) ) ;
#13836=LINE ( 'NONE', #5852, #12895 ) ;
#13841=CARTESIAN_POINT ( 'NONE',  ( -5.450524252594506791, 38.86762122992237067, 10.42016860233466247 ) ) ;
#13847=CARTESIAN_POINT ( 'NONE',  ( 3.694956938997175477, 38.77026726007181878, 13.37932843446066045 ) ) ;
#13849=CARTESIAN_POINT ( 'NONE',  ( 1.999999999999998224, 26.66874999877097352, 12.46410161513774817 ) ) ;
#13855=VECTOR ( 'NONE', #11700, 1000.000000000000000 ) ;
#13860=CARTESIAN_POINT ( 'NONE',  ( 7.437084071668728555E-15, 27.13750000000000639, 12.99999999999999112 ) ) ;
#13864=CARTESIAN_POINT ( 'NONE',  ( -3.756430356249996105, 27.65312499938548996, 11.16877607737301226 ) ) ;
#13883=PLANE ( 'NONE',  #121 ) ;
#13892=VERTEX_POINT ( 'NONE', #398 ) ;
#13895=DIRECTION ( 'NONE',  ( -0.000000000000000000, -1.000000000000000000, -0.000000000000000000 ) ) ;
#13896=ADVANCED_FACE ( 'NONE', ( #10446 ), #9933, .T. ) ;
#13902=CARTESIAN_POINT ( 'NONE',  ( 4.000000000000001776, 25.00000000000000000, 8.999999999999992895 ) ) ;
#13903=CYLINDRICAL_SURFACE ( 'NONE', #12927, 6.000000000000000888 ) ;
#13906=AXIS2_PLACEMENT_3D ( 'NONE', #2989, #1279, #11340 ) ;
#13916=CARTESIAN_POINT ( 'NONE',  ( 1.999999999999998224, 29.36874999877097636, 12.46410161513774817 ) ) ;
#13927=CARTESIAN_POINT ( 'NONE',  ( -1.999999999999996669, 26.14374999877097494, 12.46410161513774639 ) ) ;
#13929=CARTESIAN_POINT ( 'NONE',  ( 0.4995657836784084815, 38.49999999999999289, 14.97916666666666075 ) ) ;
#13931=CARTESIAN_POINT ( 'NONE',  ( -3.756430356249997882, 28.51562499938548711, 8.999999999999992895 ) ) ;
#13934=FACE_OUTER_BOUND ( 'NONE', #21659, .T. ) ;
#13935=CARTESIAN_POINT ( 'NONE',  ( 4.000000000000003553, 28.15000000000000924, 8.999999999999992895 ) ) ;
#13950=CARTESIAN_POINT ( 'NONE',  ( -1.878215178124999829, 27.80312499938548854, 12.25316411605951927 ) ) ;
#13953=CARTESIAN_POINT ( 'NONE',  ( 3.469446951953614189E-15, 31.50000000000000000, 8.999999999999992895 ) ) ;
#13958=CARTESIAN_POINT ( 'NONE',  ( -1.878215178124994722, 26.64062499938549067, 5.746835883940462963 ) ) ;
#13960=APPLICATION_CONTEXT ( 'automotive_design' ) ;
#13968=CARTESIAN_POINT ( 'NONE',  ( 3.469446951953614189E-15, 35.50000000000000711, 4.999999999999992006 ) ) ;
#13969=FACE_OUTER_BOUND ( 'NONE', #9851, .T. ) ;
#13975=CARTESIAN_POINT ( 'NONE',  ( 5.362893858306010841, 38.69544407654356633, 6.779098926265750613 ) ) ;
#13982=PLANE ( 'NONE',  #21518 ) ;
#13984=CARTESIAN_POINT ( 'NONE',  ( 2.000000000000005329, 28.61874999877097281, 5.535898384862238508 ) ) ;
#13990=CARTESIAN_POINT ( 'NONE',  ( -3.034740478393307406, 38.86679461760645182, 13.74602361519018068 ) ) ;
#13992=CARTESIAN_POINT ( 'NONE',  ( 3.756430356250003211, 27.39062499938548711, 8.999999999999992895 ) ) ;
#13999=CARTESIAN_POINT ( 'NONE',  ( 3.469446951953614189E-15, 35.50000000000000711, 4.999999999999992006 ) ) ;
#14022=EDGE_LOOP ( 'NONE', ( #13024, #7643, #2487, #11236 ) ) ;
#14029=CARTESIAN_POINT ( 'NONE',  ( 4.000000000000002665, 25.86250000000000071, 11.30940107675849760 ) ) ;
#14042=CARTESIAN_POINT ( 'NONE',  ( -2.003086131649545506E-15, 26.49062499938548143, 13.33755215474602984 ) ) ;
#14055=CARTESIAN_POINT ( 'NONE',  ( 0.07783014623661463349, 38.99999999999949551, 3.499999999999539479 ) ) ;
#14057=CARTESIAN_POINT ( 'NONE',  ( 4.000000000000001776, 29.50000000000000711, 8.999999999999992895 ) ) ;
#14058=CARTESIAN_POINT ( 'NONE',  ( 5.532151103383247559, 34.50000000000000000, 11.32277940608563149 ) ) ;
#14064=LINE ( 'NONE', #6836, #20571 ) ;
#14072=CARTESIAN_POINT ( 'NONE',  ( 0.000000000000000000, 27.84062499938549351, 13.33755215474603162 ) ) ;
#14073=ORIENTED_EDGE ( 'NONE', *, *, #4824, .F. ) ;
#14081=CARTESIAN_POINT ( 'NONE',  ( 3.756430356250004543, 27.87812499938548783, 6.831223922626973533 ) ) ;
#14092=CARTESIAN_POINT ( 'NONE',  ( 7.437084071668728555E-15, 26.63124999877097565, 12.99999999999999112 ) ) ;
#14104=CARTESIAN_POINT ( 'NONE',  ( 1.071796769724494114, 26.83615380933863648, 4.999999999999989342 ) ) ;
#14116=CARTESIAN_POINT ( 'NONE',  ( 6.009258394948636914E-15, 26.26562499938548356, 4.662447845253954171 ) ) ;
#14117=AXIS2_PLACEMENT_3D ( 'NONE', #8022, #16008, #23974 ) ;
#14118=CARTESIAN_POINT ( 'NONE',  ( 1.878215178125006934, 27.91562499938549280, 5.746835883940462963 ) ) ;
#14123=LINE ( 'NONE', #4435, #2541 ) ;
#14133=CARTESIAN_POINT ( 'NONE',  ( 1.071796769724496334, 28.18615380933863435, 4.999999999999992895 ) ) ;
#14147=ADVANCED_FACE ( 'NONE', ( #21298 ), #7813, .F. ) ;
#14148=ORIENTED_EDGE ( 'NONE', *, *, #11274, .T. ) ;
#14166=CARTESIAN_POINT ( 'NONE',  ( 2.003086131649545506E-15, 25.59062499938548996, 13.33755215474602984 ) ) ;
#14180=CARTESIAN_POINT ( 'NONE',  ( -0.4949451094549311425, 38.61079987549954495, 14.86836679116710691 ) ) ;
#14186=CARTESIAN_POINT ( 'NONE',  ( 2.000000000000000000, 29.42500000000000426, 12.46410161513774817 ) ) ;
#14203=CARTESIAN_POINT ( 'NONE',  ( -1.878215178124994722, 26.75312499938549138, 5.746835883940462963 ) ) ;
#14208=CARTESIAN_POINT ( 'NONE',  ( 4.000000000000002665, 27.21250000000000568, 11.30940107675849760 ) ) ;
#14213=CARTESIAN_POINT ( 'NONE',  ( 3.756430356250004543, 28.70312499938549067, 11.16877607737301226 ) ) ;
#14226=DIRECTION ( 'NONE',  ( -0.000000000000000000, -1.000000000000000000, -0.000000000000000000 ) ) ;
#14235=CIRCLE ( 'NONE', #6297, 6.000000000000000000 ) ;
#14244=CARTESIAN_POINT ( 'NONE',  ( 5.706339097770919189, 29.50000000000000000, 7.145898033750285983 ) ) ;
#14249=ORIENTED_EDGE ( 'NONE', *, *, #25156, .T. ) ;
#14252=CARTESIAN_POINT ( 'NONE',  ( 3.756430356250003211, 25.70312499938548356, 8.999999999999992895 ) ) ;
#14257=EDGE_CURVE ( 'NONE', #14559, #8133, #13276, .T. ) ;
#14264=DIRECTION ( 'NONE',  ( -0.000000000000000000, -1.000000000000000000, -0.000000000000000000 ) ) ;
#14274=CARTESIAN_POINT ( 'NONE',  ( 3.469446951953614189E-15, 38.49999999999999289, 8.999999999999992895 ) ) ;
#14312=CARTESIAN_POINT ( 'NONE',  ( 6.009258394948636914E-15, 27.61562499938548854, 4.662447845253954171 ) ) ;
#14315=VERTEX_POINT ( 'NONE', #14744 ) ;
#14325=CIRCLE ( 'NONE', #13906, 6.000000000000000000 ) ;
#14334=CARTESIAN_POINT ( 'NONE',  ( -0.4860084296119258074, 38.61007524145222192, 3.130138664374117585 ) ) ;
#14340=ORIENTED_EDGE ( 'NONE', *, *, #22902, .T. ) ;
#14343=CARTESIAN_POINT ( 'NONE',  ( 1.878215178124999829, 28.32812499938549422, 12.25316411605952283 ) ) ;
#14352=CARTESIAN_POINT ( 'NONE',  ( 1.878215178125003382, 27.01562499938548711, 5.746835883940462963 ) ) ;
#14368=CARTESIAN_POINT ( 'NONE',  ( 5.218530426542799638, 39.00437929243753388, 7.275652536849361418 ) ) ;
#14372=COLOUR_RGB ( '',0.8941176470588234615, 0.8941176470588234615, 0.8941176470588234615 ) ;
#14387=CARTESIAN_POINT ( 'NONE',  ( 1.878215178125001605, 26.52812499938548640, 12.25316411605952283 ) ) ;
#14398=FACE_OUTER_BOUND ( 'NONE', #2221, .T. ) ;
#14409=ORIENTED_EDGE ( 'NONE', *, *, #14768, .F. ) ;
#14416=FACE_OUTER_BOUND ( 'NONE', #14022, .T. ) ;
#14432=CARTESIAN_POINT ( 'NONE',  ( 1.878215178125005158, 28.47812499938549280, 5.746835883940462963 ) ) ;
#14435=ORIENTED_EDGE ( 'NONE', *, *, #19056, .T. ) ;
#14445=B_SPLINE_CURVE_WITH_KNOTS ( 'NONE', 3,
 ( #1557, #5611, #18039, #15943, #13847, #11993, #13592, #124, #21686, #15804, #25486, #15683, #17893, #19846, #21559, #23651 ),
 .UNSPECIFIED., .F., .F.,
 ( 4, 2, 2, 2, 2, 2, 2, 4 ),
 ( 2.789812634829633135E-07, 0.0002322844908106884518, 0.0004642900003578939055, 0.0006962955099050993591, 0.0009283010194523048670, 0.001160306528999510483, 0.001392312038546715883, 0.001856323057641126898 ),
 .UNSPECIFIED. ) ;
#14448=DIRECTION ( 'NONE',  ( 0.000000000000000000, 0.000000000000000000, -1.000000000000000000 ) ) ;
#14451=CARTESIAN_POINT ( 'NONE',  ( 8.012344526598182026E-15, 28.71250000000000568, 4.381197846482986158 ) ) ;
#14463=CARTESIAN_POINT ( 'NONE',  ( -3.756430356249994773, 28.17812499938548854, 8.999999999999992895 ) ) ;
#14464=ORIENTED_EDGE ( 'NONE', *, *, #20276, .F. ) ;
#14470=EDGE_CURVE ( 'NONE', #17209, #7506, #1593, .T. ) ;
#14472=CARTESIAN_POINT ( 'NONE',  ( 3.756430356250002323, 27.42812499938548498, 6.831223922626973533 ) ) ;
#14476=DIRECTION ( 'NONE',  ( -0.000000000000000000, 1.000000000000000000, 0.000000000000000000 ) ) ;
#14496=CARTESIAN_POINT ( 'NONE',  ( 2.000000000000000000, 29.81874999877097210, 12.46410161513774817 ) ) ;
#14498=EDGE_CURVE ( 'NONE', #2175, #14315, #13428, .T. ) ;
#14502=FACE_OUTER_BOUND ( 'NONE', #24310, .T. ) ;
#14509=DIRECTION ( 'NONE',  ( -0.000000000000000000, -1.000000000000000000, -0.000000000000000000 ) ) ;
#14516=CARTESIAN_POINT ( 'NONE',  ( -1.999999999999998224, 27.55000000000000426, 12.46410161513774639 ) ) ;
#14517=DIRECTION ( 'NONE',  ( 3.552713678800501718E-15, 0.000000000000000000, 1.000000000000000000 ) ) ;
#14521=CARTESIAN_POINT ( 'NONE',  ( 4.000000000000002665, 27.60624999877096641, 11.30940107675849760 ) ) ;
#14527=ORIENTED_EDGE ( 'NONE', *, *, #2082, .T. ) ;
#14531=FACE_OUTER_BOUND ( 'NONE', #15537, .T. ) ;
#14533=EDGE_CURVE ( 'NONE', #17574, #11405, #5437, .T. ) ;
#14543=CARTESIAN_POINT ( 'NONE',  ( 4.143002691484658293E-15, 39.50000000000000000, 13.99999999999999289 ) ) ;
#14550=CARTESIAN_POINT ( 'NONE',  ( -1.878215178124998275, 27.35312499938548925, 12.25316411605951927 ) ) ;
#14554=DIRECTION ( 'NONE',  ( 0.000000000000000000, -1.000000000000000000, 0.000000000000000000 ) ) ;
#14559=VERTEX_POINT ( 'NONE', #3723 ) ;
#14564=EDGE_CURVE ( 'NONE', #23529, #22370, #25060, .T. ) ;
#14568=CARTESIAN_POINT ( 'NONE',  ( -1.999999999999998224, 28.90000000000000924, 12.46410161513774639 ) ) ;
#14572=( BOUNDED_CURVE ( )  B_SPLINE_CURVE ( 2, ( #18583, #16498, #20267, #14521, #18837, #24462, #409, #18316, #2750 ),
 .UNSPECIFIED., .F., .F. ) 
 B_SPLINE_CURVE_WITH_KNOTS ( ( 3, 2, 2, 2, 3 ),
 ( 0.4750000000000000333, 0.4833333333333333370, 0.5000000000000000000, 0.5166666666666667185, 0.5250000000000000222 ),
 .UNSPECIFIED. ) 
 CURVE ( )  GEOMETRIC_REPRESENTATION_ITEM ( )  RATIONAL_B_SPLINE_CURVE ( ( 0.9330127018922194093, 0.9330127018922196314, 1.000000000000000000, 0.8660254037844387076, 1.000000000000000000, 0.8660254037844387076, 1.000000000000000000, 0.9330127018922194093, 0.9330127018922194093 ) ) 
 REPRESENTATION_ITEM ( '' )  );
#14585=CARTESIAN_POINT ( 'NONE',  ( 3.756430356250004099, 29.71562499938548996, 11.16877607737301403 ) ) ;
#14592=CARTESIAN_POINT ( 'NONE',  ( 4.006172263299091013E-15, 28.17812499938548498, 13.33755215474602984 ) ) ;
#14597=CARTESIAN_POINT ( 'NONE',  ( -3.756430356249996105, 25.77812499938548640, 6.831223922626973533 ) ) ;
#14640=CARTESIAN_POINT ( 'NONE',  ( -3.068646161593051591, 38.57519691277454399, 3.931793986884403402 ) ) ;
#14642=CARTESIAN_POINT ( 'NONE',  ( 3.469446951953614189E-15, 38.49999999999999289, 8.999999999999992895 ) ) ;
#14682=CARTESIAN_POINT ( 'NONE',  ( -1.999999999999993117, 28.69374999877097210, 5.535898384862237620 ) ) ;
#14687=EDGE_CURVE ( 'NONE', #21027, #24856, #22810, .T. ) ;
#14692=CARTESIAN_POINT ( 'NONE',  ( -3.756430356249996105, 27.76562499938549422, 11.16877607737301226 ) ) ;
#14703=ORIENTED_EDGE ( 'NONE', *, *, #23772, .F. ) ;
#14709=CARTESIAN_POINT ( 'NONE',  ( -3.999999999999996447, 26.57500000000000639, 8.999999999999992895 ) ) ;
#14715=CYLINDRICAL_SURFACE ( 'NONE', #25791, 4.000000000000000000 ) ;
#14718=CARTESIAN_POINT ( 'NONE',  ( 4.000000000000003553, 26.29374999877097352, 8.999999999999992895 ) ) ;
#14734=CARTESIAN_POINT ( 'NONE',  ( 0.4995657836784154204, 34.50000000000000000, 3.020833333333324600 ) ) ;
#14735=CARTESIAN_POINT ( 'NONE',  ( -1.878215178124998275, 25.44062499938549138, 12.25316411605951927 ) ) ;
#14738=CARTESIAN_POINT ( 'NONE',  ( 1.878215178125001605, 25.96562499938548996, 12.25316411605952283 ) ) ;
#14744=CARTESIAN_POINT ( 'NONE',  ( 4.000000000000001776, 29.89374999877097139, 8.999999999999992895 ) ) ;
#14768=EDGE_CURVE ( 'NONE', #21315, #12001, #13836, .T. ) ;
#14770=CARTESIAN_POINT ( 'NONE',  ( 3.756430356250001434, 27.50312499938548783, 8.999999999999992895 ) ) ;
#14779=DIRECTION ( 'NONE',  ( 0.000000000000000000, -1.000000000000000000, 0.000000000000000000 ) ) ;
#14800=VERTEX_POINT ( 'NONE', #23518 ) ;
#14823=CARTESIAN_POINT ( 'NONE',  ( 2.003086131649545506E-15, 27.39062499938549067, 13.33755215474602984 ) ) ;
#14828=ORIENTED_EDGE ( 'NONE', *, *, #1500, .T. ) ;
#14829=DIRECTION ( 'NONE',  ( -0.000000000000000000, -1.000000000000000000, -0.000000000000000000 ) ) ;
#14846=CARTESIAN_POINT ( 'NONE',  ( 4.000000000000005329, 25.88124999877096855, 6.690598923241489970 ) ) ;
#14851=CARTESIAN_POINT ( 'NONE',  ( 3.469446951953614189E-15, 39.50000000000000000, 3.999999999999991562 ) ) ;
#14855=DIRECTION ( 'NONE',  ( 0.000000000000000000, 0.000000000000000000, -1.000000000000000000 ) ) ;
#14856=LINE ( 'NONE', #20606, #12148 ) ;
#14863=CARTESIAN_POINT ( 'NONE',  ( 8.012344526598182026E-15, 28.85312499938549280, 4.662447845253954171 ) ) ;
#14880=DIRECTION ( 'NONE',  ( 0.000000000000000000, 1.000000000000000000, 0.000000000000000000 ) ) ;
#14888=EDGE_LOOP ( 'NONE', ( #13626, #24071, #25665, #24201 ) ) ;
#14891=CARTESIAN_POINT ( 'NONE',  ( 1.878215178125005158, 28.47812499938549280, 5.746835883940462963 ) ) ;
#14915=ADVANCED_FACE ( 'NONE', ( #13969 ), #14715, .T. ) ;
#14943=EDGE_CURVE ( 'NONE', #19496, #16533, #24146, .T. ) ;
#14944=ORIENTED_EDGE ( 'NONE', *, *, #389, .F. ) ;
#14966=CARTESIAN_POINT ( 'NONE',  ( -3.999999999999998224, 28.31874999877097210, 8.999999999999992895 ) ) ;
#14973=CARTESIAN_POINT ( 'NONE',  ( 3.756430356250004099, 28.89062499938549067, 6.831223922626973533 ) ) ;
#14979=AXIS2_PLACEMENT_3D ( 'NONE', #9900, #5986, #17886 ) ;
#14983=CARTESIAN_POINT ( 'NONE',  ( -2.003086131649545506E-15, 26.37812499938548427, 13.33755215474603162 ) ) ;
#14985=CARTESIAN_POINT ( 'NONE',  ( 0.000000000000000000, 28.62812499938549138, 13.33755215474602984 ) ) ;
#14986=VECTOR ( 'NONE', #1129, 1000.000000000000000 ) ;
#14987=CARTESIAN_POINT ( 'NONE',  ( 2.000000000000005329, 25.52500000000000568, 5.535898384862238508 ) ) ;
#15010=CARTESIAN_POINT ( 'NONE',  ( 3.469446951953614189E-15, 39.50000000000000000, 3.999999999999991562 ) ) ;
#15013=ORIENTED_EDGE ( 'NONE', *, *, #7648, .T. ) ;
#15018=CARTESIAN_POINT ( 'NONE',  ( 3.756430356250004987, 27.95312499938548711, 8.999999999999992895 ) ) ;
#15020=VECTOR ( 'NONE', #20323, 1000.000000000000000 ) ;
#15038=CIRCLE ( 'NONE', #3749, 0.5000000000000004441 ) ;
#15042=FACE_OUTER_BOUND ( 'NONE', #22369, .T. ) ;
#15044=CARTESIAN_POINT ( 'NONE',  ( -5.357848403820182348, 38.93885650637880502, 7.509366431266231601 ) ) ;
#15046=VERTEX_POINT ( 'NONE', #19134 ) ;
#15053=DIRECTION ( 'NONE',  ( 0.000000000000000000, -1.000000000000000000, -0.000000000000000000 ) ) ;
#15099=EDGE_CURVE ( 'NONE', #7296, #19084, #15230, .T. ) ;
#15107=CARTESIAN_POINT ( 'NONE',  ( 4.000000000000002665, 28.13124999877096855, 6.690598923241489970 ) ) ;
#15113=LINE ( 'NONE', #14851, #12114 ) ;
#15123=CARTESIAN_POINT ( 'NONE',  ( 1.878215178125006934, 29.26562499938549067, 5.746835883940462963 ) ) ;
#15125=CARTESIAN_POINT ( 'NONE',  ( -1.878215178124998275, 25.89062499938549067, 12.25316411605951927 ) ) ;
#15126=LINE ( 'NONE', #7515, #25534 ) ;
#15127=CARTESIAN_POINT ( 'NONE',  ( 0.000000000000000000, 29.52812499938548640, 13.33755215474602984 ) ) ;
#15134=VECTOR ( 'NONE', #2816, 1000.000000000000000 ) ;
#15147=LINE ( 'NONE', #16853, #13389 ) ;
#15153=ORIENTED_EDGE ( 'NONE', *, *, #5958, .T. ) ;
#15161=CARTESIAN_POINT ( 'NONE',  ( 0.000000000000000000, 28.74062499938548854, 13.33755215474602984 ) ) ;
#15197=DIRECTION ( 'NONE',  ( 0.000000000000000000, -1.000000000000000000, 0.000000000000000000 ) ) ;
#15206=CARTESIAN_POINT ( 'NONE',  ( -3.999999999999999112, 25.18750000000000711, 6.690598923241487306 ) ) ;
#15214=VERTEX_POINT ( 'NONE', #12055 ) ;
#15217=DIRECTION ( 'NONE',  ( -0.000000000000000000, -1.000000000000000000, -0.000000000000000000 ) ) ;
#15230=LINE ( 'NONE', #5407, #23341 ) ;
#15234=CARTESIAN_POINT ( 'NONE',  ( 4.000000000000007105, 26.78124999877097423, 6.690598923241489970 ) ) ;
#15236=EDGE_LOOP ( 'NONE', ( #16047, #2810, #7129, #6548 ) ) ;
#15240=EDGE_CURVE ( 'NONE', #4730, #17275, #17471, .T. ) ;
#15244=DIRECTION ( 'NONE',  ( 0.000000000000000000, 0.000000000000000000, -1.000000000000000000 ) ) ;
#15250=CARTESIAN_POINT ( 'NONE',  ( 3.756430356250000546, 29.15312499938548996, 11.16877607737301226 ) ) ;
#15257=CARTESIAN_POINT ( 'NONE',  ( -4.648177544792955347E-16, 27.08124999877097139, 12.99999999999999289 ) ) ;
#15260=( BOUNDED_CURVE ( )  B_SPLINE_CURVE ( 2, ( #13251, #17702, #13386, #17320, #11666, #3686, #21608, #19390, #7243 ),
 .UNSPECIFIED., .F., .F. ) 
 B_SPLINE_CURVE_WITH_KNOTS ( ( 3, 2, 2, 2, 3 ),
 ( 0.1250000000000000000, 0.1333333333333333315, 0.1499999999999999944, 0.1666666666666666574, 0.1749999999999999889 ),
 .UNSPECIFIED. ) 
 CURVE ( )  GEOMETRIC_REPRESENTATION_ITEM ( )  RATIONAL_B_SPLINE_CURVE ( ( 0.9330127018922194093, 0.9330127018922194093, 1.000000000000000000, 0.8660254037844387076, 1.000000000000000000, 0.8660254037844387076, 1.000000000000000000, 0.9330127018922194093, 0.9330127018922194093 ) ) 
 REPRESENTATION_ITEM ( '' )  );
#15280=CARTESIAN_POINT ( 'NONE',  ( 4.006172263299091013E-15, 28.96562499938548996, 4.662447845253954171 ) ) ;
#15300=DIRECTION ( 'NONE',  ( -3.552713678800501718E-15, 0.000000000000000000, 1.000000000000000000 ) ) ;
#15320=DIRECTION ( 'NONE',  ( -0.000000000000000000, -1.000000000000000000, -0.000000000000000000 ) ) ;
#15323=CARTESIAN_POINT ( 'NONE',  ( -5.840899737312982509, 38.49999999999999289, 7.627451181685283466 ) ) ;
#15324=DIRECTION ( 'NONE',  ( -0.000000000000000000, -1.000000000000000000, -0.000000000000000000 ) ) ;
#15329=EDGE_CURVE ( 'NONE', #21027, #6423, #3834, .T. ) ;
#15348=ORIENTED_EDGE ( 'NONE', *, *, #12700, .F. ) ;
#15350=CARTESIAN_POINT ( 'NONE',  ( -4.000000000000000000, 27.41874999877096997, 8.999999999999992895 ) ) ;
#15352=ORIENTED_EDGE ( 'NONE', *, *, #5782, .F. ) ;
#15357=ORIENTED_EDGE ( 'NONE', *, *, #18499, .T. ) ;
#15359=EDGE_CURVE ( 'NONE', #21315, #13062, #24531, .T. ) ;
#15365=CARTESIAN_POINT ( 'NONE',  ( 1.878215178125003382, 27.46562499938548996, 5.746835883940462963 ) ) ;
#15366=EDGE_CURVE ( 'NONE', #19882, #17641, #18484, .T. ) ;
#15369=CARTESIAN_POINT ( 'NONE',  ( -3.756430356249997882, 28.51562499938548711, 8.999999999999992895 ) ) ;
#15373=DIRECTION ( 'NONE',  ( 0.000000000000000000, 0.000000000000000000, 1.000000000000000000 ) ) ;
#15395=VERTEX_POINT ( 'NONE', #4350 ) ;
#15397=CARTESIAN_POINT ( 'NONE',  ( 1.878215178125003382, 29.37812499938548783, 5.746835883940462963 ) ) ;
#15405=( NAMED_UNIT ( * ) PLANE_ANGLE_UNIT ( ) SI_UNIT ( $, .RADIAN. ) );
#15409=CARTESIAN_POINT ( 'NONE',  ( 4.000000000000002665, 26.76250000000000284, 11.30940107675849760 ) ) ;
#15437=CARTESIAN_POINT ( 'NONE',  ( -1.878215178124998275, 25.44062499938549138, 12.25316411605951927 ) ) ;
#15447=CARTESIAN_POINT ( 'NONE',  ( 4.000000000000001776, 29.69687499938548925, 8.999999999999992895 ) ) ;
#15458=AXIS2_PLACEMENT_3D ( 'NONE', #8569, #8302, #24001 ) ;
#15463=ORIENTED_EDGE ( 'NONE', *, *, #22508, .T. ) ;
#15489=EDGE_LOOP ( 'NONE', ( #2299, #16562, #14340, #3810 ) ) ;
#15490=CARTESIAN_POINT ( 'NONE',  ( 2.000000000000000000, 28.01874999877097139, 12.46410161513774817 ) ) ;
#15495=CIRCLE ( 'NONE', #16310, 6.000000000000000000 ) ;
#15497=DIRECTION ( 'NONE',  ( 0.000000000000000000, 0.000000000000000000, 1.000000000000000000 ) ) ;
#15507=CARTESIAN_POINT ( 'NONE',  ( 1.878215178125003382, 27.01562499938548711, 5.746835883940462963 ) ) ;
#15508=VECTOR ( 'NONE', #14509, 1000.000000000000000 ) ;
#15510=CARTESIAN_POINT ( 'NONE',  ( 8.012344526598182026E-15, 26.91250000000000497, 4.381197846482986158 ) ) ;
#15537=EDGE_LOOP ( 'NONE', ( #9572, #23318, #15153, #13307 ) ) ;
#15538=ORIENTED_EDGE ( 'NONE', *, *, #20182, .T. ) ;
#15540=AXIS2_PLACEMENT_3D ( 'NONE', #6273, #14264, #7842 ) ;
#15541=CARTESIAN_POINT ( 'NONE',  ( -3.756430356249996105, 26.22812499938548569, 6.831223922626973533 ) ) ;
#15580=( BOUNDED_CURVE ( )  B_SPLINE_CURVE ( 2, ( #22358, #2622, #6533, #18578, #4442, #12415, #14516, #2482, #10450 ),
 .UNSPECIFIED., .F., .F. ) 
 B_SPLINE_CURVE_WITH_KNOTS ( ( 3, 2, 2, 2, 3 ),
 ( 0.5250000000000000222, 0.5333333333333333259, 0.5500000000000000444, 0.5666666666666666519, 0.5750000000000000666 ),
 .UNSPECIFIED. ) 
 CURVE ( )  GEOMETRIC_REPRESENTATION_ITEM ( )  RATIONAL_B_SPLINE_CURVE ( ( 0.9330127018922194093, 0.9330127018922194093, 1.000000000000000000, 0.8660254037844387076, 1.000000000000000000, 0.8660254037844387076, 1.000000000000000000, 0.9330127018922189652, 0.9330127018922194093 ) ) 
 REPRESENTATION_ITEM ( '' )  );
#15592=FACE_OUTER_BOUND ( 'NONE', #20705, .T. ) ;
#15594=LINE ( 'NONE', #719, #8767 ) ;
#15614=CARTESIAN_POINT ( 'NONE',  ( -3.999999999999999112, 27.45624999877097139, 11.30940107675849404 ) ) ;
#15622=CARTESIAN_POINT ( 'NONE',  ( -3.756430356249996105, 25.96562499938548996, 11.16877607737301226 ) ) ;
#15630=ORIENTED_EDGE ( 'NONE', *, *, #144, .T. ) ;
#15636=CARTESIAN_POINT ( 'NONE',  ( -1.878215178124996498, 27.54062499938548569, 5.746835883940462963 ) ) ;
#15639=CARTESIAN_POINT ( 'NONE',  ( 4.000000000000001776, 27.70000000000000639, 8.999999999999992895 ) ) ;
#15640=EDGE_CURVE ( 'NONE', #18698, #4270, #21141, .T. ) ;
#15644=CARTESIAN_POINT ( 'NONE',  ( -4.648177544792955347E-16, 26.85624999877096997, 4.999999999999991118 ) ) ;
#15653=CARTESIAN_POINT ( 'NONE',  ( 5.577813053751546416E-15, 25.95624999877097139, 4.999999999999992006 ) ) ;
#15666=CARTESIAN_POINT ( 'NONE',  ( 3.756430356250004987, 29.75312499938549138, 8.999999999999992895 ) ) ;
#15669=CARTESIAN_POINT ( 'NONE',  ( 5.577813053751546416E-15, 28.20624999877096784, 4.999999999999992006 ) ) ;
#15671=CARTESIAN_POINT ( 'NONE',  ( 2.000000000000005329, 28.67500000000000426, 5.535898384862238508 ) ) ;
#15672=CARTESIAN_POINT ( 'NONE',  ( 2.000000000000007105, 29.51874999877097139, 5.535898384862238508 ) ) ;
#15683=CARTESIAN_POINT ( 'NONE',  ( 3.052426026682831139, 38.91217497027906802, 13.68084836822773553 ) ) ;
#15689=VERTEX_POINT ( 'NONE', #15323 ) ;
#15692=ORIENTED_EDGE ( 'NONE', *, *, #15924, .T. ) ;
#15703=DIRECTION ( 'NONE',  ( 0.000000000000000000, 0.000000000000000000, 1.000000000000000000 ) ) ;
#15710=CARTESIAN_POINT ( 'NONE',  ( 4.000000000000003553, 26.29374999877097352, 8.999999999999992895 ) ) ;
#15712=DIRECTION ( 'NONE',  ( 0.000000000000000000, 1.000000000000000000, 0.000000000000000000 ) ) ;
#15717=DIRECTION ( 'NONE',  ( -0.000000000000000000, -1.000000000000000000, -0.000000000000000000 ) ) ;
#15744=CARTESIAN_POINT ( 'NONE',  ( 4.000000000000005329, 29.44374999877097210, 8.999999999999992895 ) ) ;
#15750=VERTEX_POINT ( 'NONE', #23678 ) ;
#15752=ORIENTED_EDGE ( 'NONE', *, *, #15640, .T. ) ;
#15755=CARTESIAN_POINT ( 'NONE',  ( -1.878215178124999829, 27.69062499938549138, 12.25316411605951927 ) ) ;
#15757=CARTESIAN_POINT ( 'NONE',  ( 4.000000000000005329, 27.25000000000000355, 8.999999999999992895 ) ) ;
#15770=ORIENTED_EDGE ( 'NONE', *, *, #17524, .T. ) ;
#15774=ORIENTED_EDGE ( 'NONE', *, *, #10685, .T. ) ;
#15781=CARTESIAN_POINT ( 'NONE',  ( 3.469446951953614189E-15, 35.50000000000000711, 8.999999999999992895 ) ) ;
#15782=CARTESIAN_POINT ( 'NONE',  ( 3.756430356250000546, 29.26562499938549067, 11.16877607737301226 ) ) ;
#15784=( BOUNDED_CURVE ( )  B_SPLINE_CURVE ( 2, ( #3202, #11308, #10780, #11051, #24921, #6745, #16688, #18774, #14735, #13028, #23213, #19032, #24659, #23098, #16831, #21008, #1114, #25048, #7137, #21249, #15125, #10920, #13158, #11170, #5046, #2956, #4793, #8979, #5297, #17217, #13277, #6999, #1244, #14983, #9228, #25187, #3330, #22712, #12768, #20739, #2817, #864, #8844, #24795, #6877, #4909, #3712, #5807, #25426, #5946, #15507, #7387, #25693, #17456, #19801, #19287, #21899, #25567, #17723, #13415, #13793, #11443, #15365, #3982, #15636, #25815, #23603, #9478, #15755, #1386, #3590, #1507, #1901, #19670, #1776, #9361, #19530, #11694, #17344, #5562, #7650, #3470, #15888, #21510, #3853, #7513, #9864, #9743, #23474, #13545, #13931, #7776, #25309, #11562, #21631, #23860, #1631, #9606, #21769, #23337, #17591, #5427, #5681, #21390, #23718, #13660, #11831, #19414, #17847, #7898, #2402, #8558, #23988, #8169, #10239, #69, #6071, #16274, #10124, #4100, #16148 ),
 .UNSPECIFIED., .F., .T. ) 
 B_SPLINE_CURVE_WITH_KNOTS ( ( 3, 2, 2, 2, 2, 2, 2, 2, 2, 2, 2, 2, 2, 2, 2, 2, 2, 2, 2, 2, 2, 2, 2, 2, 2, 2, 2, 2, 2, 2, 2, 2, 2, 2, 2, 2, 2, 2, 2, 2, 2, 2, 2, 2, 2, 2, 2, 2, 2, 2, 2, 2, 2, 2, 2, 2, 2, 2, 2, 2, 3 ),
 ( 0.000000000000000000, 0.01666666666666666644, 0.03333333333333333287, 0.05000000000000000278, 0.06666666666666666574, 0.08333333333333332871, 0.1000000000000000056, 0.1166666666666666685, 0.1333333333333333315, 0.1499999999999999944, 0.1666666666666666574, 0.1833333333333333204, 0.2000000000000000111, 0.2166666666666666741, 0.2333333333333333370, 0.2500000000000000000, 0.2666666666666666630, 0.2833333333333333259, 0.2999999999999999889, 0.3166666666666666519, 0.3333333333333333148, 0.3499999999999999778, 0.3666666666666666408, 0.3833333333333333592, 0.4000000000000000222, 0.4166666666666666852, 0.4333333333333333481, 0.4500000000000000111, 0.4666666666666666741, 0.4833333333333333370, 0.5000000000000000000, 0.5166666666666667185, 0.5333333333333333259, 0.5500000000000000444, 0.5666666666666666519, 0.5833333333333333703, 0.5999999999999999778, 0.6166666666666666963, 0.6333333333333333037, 0.6500000000000000222, 0.6666666666666666297, 0.6833333333333333481, 0.6999999999999999556, 0.7166666666666666741, 0.7333333333333332815, 0.7500000000000000000, 0.7666666666666667185, 0.7833333333333333259, 0.8000000000000000444, 0.8166666666666666519, 0.8333333333333333703, 0.8499999999999999778, 0.8666666666666666963, 0.8833333333333333037, 0.9000000000000000222, 0.9166666666666666297, 0.9333333333333333481, 0.9499999999999999556, 0.9666666666666666741, 0.9833333333333332815, 1.000000000000000000 ),
 .UNSPECIFIED. ) 
 CURVE ( )  GEOMETRIC_REPRESENTATION_ITEM ( )  RATIONAL_B_SPLINE_CURVE ( ( 1.000000000000000000, 0.8660254037844387076, 1.000000000000000000, 0.8660254037844387076, 1.000000000000000000, 0.8660254037844387076, 1.000000000000000000, 0.8660254037844387076, 1.000000000000000000, 0.8660254037844387076, 1.000000000000000000, 0.8660254037844387076, 1.000000000000000000, 0.8660254037844387076, 1.000000000000000000, 0.8660254037844387076, 1.000000000000000000, 0.8660254037844387076, 1.000000000000000000, 0.8660254037844387076, 1.000000000000000000, 0.8660254037844387076, 1.000000000000000000, 0.8660254037844387076, 1.000000000000000000, 0.8660254037844387076, 1.000000000000000000, 0.8660254037844387076, 1.000000000000000000, 0.8660254037844387076, 1.000000000000000000, 0.8660254037844387076, 1.000000000000000000, 0.8660254037844387076, 1.000000000000000000, 0.8660254037844387076, 1.000000000000000000, 0.8660254037844387076, 1.000000000000000000, 0.8660254037844387076, 1.000000000000000000, 0.8660254037844387076, 1.000000000000000000, 0.8660254037844387076, 1.000000000000000000, 0.8660254037844387076, 1.000000000000000000, 0.8660254037844387076, 1.000000000000000000, 0.8660254037844387076, 1.000000000000000000, 0.8660254037844387076, 1.000000000000000000, 0.8660254037844387076, 1.000000000000000000, 0.8660254037844387076, 1.000000000000000000, 0.8660254037844387076, 1.000000000000000000, 0.8660254037844387076, 1.000000000000000000, 0.8660254037844387076, 1.000000000000000000, 0.8660254037844387076, 1.000000000000000000, 0.8660254037844387076, 1.000000000000000000, 0.8660254037844387076, 1.000000000000000000, 0.8660254037844387076, 1.000000000000000000, 0.8660254037844387076, 1.000000000000000000, 0.8660254037844387076, 1.000000000000000000, 0.8660254037844387076, 1.000000000000000000, 0.8660254037844387076, 1.000000000000000000, 0.8660254037844387076, 1.000000000000000000, 0.8660254037844387076, 1.000000000000000000, 0.8660254037844387076, 1.000000000000000000, 0.8660254037844387076, 1.000000000000000000, 0.8660254037844387076, 1.000000000000000000, 0.8660254037844387076, 1.000000000000000000, 0.8660254037844387076, 1.000000000000000000, 0.8660254037844387076, 1.000000000000000000, 0.8660254037844387076, 1.000000000000000000, 0.8660254037844387076, 1.000000000000000000, 0.8660254037844387076, 1.000000000000000000, 0.8660254037844387076, 1.000000000000000000, 0.8660254037844387076, 1.000000000000000000, 0.8660254037844387076, 1.000000000000000000, 0.8660254037844387076, 1.000000000000000000, 0.8660254037844387076, 1.000000000000000000, 0.8660254037844387076, 1.000000000000000000, 0.8660254037844387076, 1.000000000000000000, 0.8660254037844387076, 1.000000000000000000, 0.8660254037844387076, 1.000000000000000000, 0.8660254037844387076, 1.000000000000000000 ) ) 
 REPRESENTATION_ITEM ( '' )  );
#15785=CARTESIAN_POINT ( 'NONE',  ( -3.999999999999996447, 28.28124999877097778, 6.690598923241487306 ) ) ;
#15788=LINE ( 'NONE', #5848, #20987 ) ;
#15798=CARTESIAN_POINT ( 'NONE',  ( -5.254586613389494509, 39.00010698140259535, 10.62610181236646056 ) ) ;
#15801=EDGE_CURVE ( 'NONE', #13892, #14800, #7730, .T. ) ;
#15804=CARTESIAN_POINT ( 'NONE',  ( 3.170271286762905927, 39.00010698140257404, 13.49491574449624665 ) ) ;
#15806=CARTESIAN_POINT ( 'NONE',  ( 3.756430356250000546, 29.26562499938549067, 11.16877607737301226 ) ) ;
#15820=CARTESIAN_POINT ( 'NONE',  ( -3.756430356249994773, 25.81562499938548783, 8.999999999999992895 ) ) ;
#15831=CARTESIAN_POINT ( 'NONE',  ( 4.000000000000001776, 27.70000000000000639, 8.999999999999992895 ) ) ;
#15841=VERTEX_POINT ( 'NONE', #25520 ) ;
#15844=CARTESIAN_POINT ( 'NONE',  ( 0.000000000000000000, 31.50000000000000000, 14.99999999999999289 ) ) ;
#15848=ORIENTED_EDGE ( 'NONE', *, *, #2469, .T. ) ;
#15861=CARTESIAN_POINT ( 'NONE',  ( 3.526711513754818395, 31.50000000000000000, 4.645898033750289535 ) ) ;
#15863=AXIS2_PLACEMENT_3D ( 'NONE', #9147, #13087, #3141 ) ;
#15871=CARTESIAN_POINT ( 'NONE',  ( -1.878215178124998275, 25.55312499938549564, 12.25316411605951927 ) ) ;
#15872=CIRCLE ( 'NONE', #22117, 6.000000000000000000 ) ;
#15888=CARTESIAN_POINT ( 'NONE',  ( 1.878215178124998275, 28.21562499938549351, 12.25316411605952283 ) ) ;
#15892=CARTESIAN_POINT ( 'NONE',  ( 0.000000000000000000, 28.03750000000001208, 13.61880215351699874 ) ) ;
#15894=FACE_OUTER_BOUND ( 'NONE', #25172, .T. ) ;
#15896=AXIS2_PLACEMENT_3D ( 'NONE', #13644, #3692, #302 ) ;
#15909=CARTESIAN_POINT ( 'NONE',  ( 1.878215178125008489, 26.22812499938548925, 5.746835883940462963 ) ) ;
#15920=CARTESIAN_POINT ( 'NONE',  ( -3.756430356249994773, 29.07812499938548711, 8.999999999999992895 ) ) ;
#15924=EDGE_CURVE ( 'NONE', #1533, #3918, #352, .T. ) ;
#15928=DIRECTION ( 'NONE',  ( -0.000000000000000000, -1.000000000000000000, -0.000000000000000000 ) ) ;
#15931=CARTESIAN_POINT ( 'NONE',  ( 1.071796769724489895, 29.35134618820331198, 12.99999999999999467 ) ) ;
#15943=CARTESIAN_POINT ( 'NONE',  ( 3.749140371009410000, 38.71721868403346178, 13.40281365441718542 ) ) ;
#15960=CARTESIAN_POINT ( 'NONE',  ( 1.878215178125006934, 26.56562499938548783, 5.746835883940462963 ) ) ;
#15975=CARTESIAN_POINT ( 'NONE',  ( 4.000000000000000888, 26.25624999877096499, 11.30940107675849760 ) ) ;
#15989=CARTESIAN_POINT ( 'NONE',  ( 5.577813053751546416E-15, 27.81250000000000355, 4.999999999999992006 ) ) ;
#16000=CARTESIAN_POINT ( 'NONE',  ( -1.071796769724485676, 27.51115380933864074, 12.99999999999999467 ) ) ;
#16008=DIRECTION ( 'NONE',  ( 0.000000000000000000, 1.000000000000000000, 0.000000000000000000 ) ) ;
#16011=CARTESIAN_POINT ( 'NONE',  ( -3.756430356249996105, 25.89062499938548356, 6.831223922626973533 ) ) ;
#16018=ORIENTED_EDGE ( 'NONE', *, *, #1500, .F. ) ;
#16019=CIRCLE ( 'NONE', #18923, 0.5000000000000004441 ) ;
#16028=CARTESIAN_POINT ( 'NONE',  ( 4.000000000000007105, 25.93750000000000711, 6.690598923241489970 ) ) ;
#16035=CARTESIAN_POINT ( 'NONE',  ( -3.611812437532109232, 38.84323238218505736, 4.645898033750475165 ) ) ;
#16046=CARTESIAN_POINT ( 'NONE',  ( -3.756430356250002323, 27.31562499938548783, 11.16877607737301048 ) ) ;
#16047=ORIENTED_EDGE ( 'NONE', *, *, #4774, .T. ) ;
#16053=CARTESIAN_POINT ( 'NONE',  ( -3.756430356249994773, 28.06562499938548783, 8.999999999999992895 ) ) ;
#16059=DIRECTION ( 'NONE',  ( 0.000000000000000000, 0.000000000000000000, 1.000000000000000000 ) ) ;
#16071=ADVANCED_FACE ( 'NONE', ( #19204 ), #8757, .T. ) ;
#16078=CARTESIAN_POINT ( 'NONE',  ( -5.264710367730059737, 38.83395867543784163, 6.905309864513818674 ) ) ;
#16080=ORIENTED_EDGE ( 'NONE', *, *, #18073, .T. ) ;
#16087=CARTESIAN_POINT ( 'NONE',  ( 3.756430356250004987, 27.84062499938548640, 8.999999999999992895 ) ) ;
#16105=CARTESIAN_POINT ( 'NONE',  ( -3.999999999999998224, 27.02500000000000213, 8.999999999999992895 ) ) ;
#16135=CARTESIAN_POINT ( 'NONE',  ( 4.000000000000001776, 29.89374999877097139, 8.999999999999992895 ) ) ;
#16146=LINE ( 'NONE', #4767, #21424 ) ;
#16148=CARTESIAN_POINT ( 'NONE',  ( 3.756430356250004987, 29.64062499938548711, 8.999999999999992895 ) ) ;
#16149=CARTESIAN_POINT ( 'NONE',  ( 0.1556054994193530883, 38.97851006807006513, 3.480354713799856725 ) ) ;
#16151=CARTESIAN_POINT ( 'NONE',  ( -1.999999999999998224, 28.45000000000000639, 12.46410161513774639 ) ) ;
#16160=CARTESIAN_POINT ( 'NONE',  ( 5.337298091574883330, 38.72260848564139479, 11.21294222745710378 ) ) ;
#16164=CARTESIAN_POINT ( 'NONE',  ( 2.003086131649545506E-15, 27.39062499938549067, 13.33755215474603162 ) ) ;
#16171=CARTESIAN_POINT ( 'NONE',  ( 3.756430356250002323, 28.32812499938549067, 6.831223922626973533 ) ) ;
#16206=CARTESIAN_POINT ( 'NONE',  ( -1.878215178124998275, 28.14062499938548711, 12.25316411605951927 ) ) ;
#16210=CARTESIAN_POINT ( 'NONE',  ( -1.071796769724490561, 28.73259618943233207, 4.999999999999995559 ) ) ;
#16244=CARTESIAN_POINT ( 'NONE',  ( 2.000000000000000000, 25.82500000000000639, 12.46410161513774817 ) ) ;
#16247=CARTESIAN_POINT ( 'NONE',  ( 3.469446951953614189E-15, 38.49999999999999289, 8.999999999999992895 ) ) ;
#16257=ORIENTED_EDGE ( 'NONE', *, *, #7399, .T. ) ;
#16259=CARTESIAN_POINT ( 'NONE',  ( -3.756430356249994329, 26.79062499938549280, 6.831223922626973533 ) ) ;
#16270=ORIENTED_EDGE ( 'NONE', *, *, #6855, .T. ) ;
#16274=CARTESIAN_POINT ( 'NONE',  ( 0.000000000000000000, 29.52812499938548640, 13.33755215474603162 ) ) ;
#16279=CARTESIAN_POINT ( 'NONE',  ( 4.000000000000005329, 29.05000000000000426, 8.999999999999992895 ) ) ;
#16296=CARTESIAN_POINT ( 'NONE',  ( 1.878215178125008489, 27.57812499938549422, 5.746835883940462963 ) ) ;
#16306=CARTESIAN_POINT ( 'NONE',  ( 2.003086131649545506E-15, 29.07812499938549067, 13.33755215474602984 ) ) ;
#16310=AXIS2_PLACEMENT_3D ( 'NONE', #2009, #17334, #15497 ) ;
#16312=CARTESIAN_POINT ( 'NONE',  ( 3.526711513754840599, 38.89679573513954125, 4.645898033750303746 ) ) ;
#16315=CIRCLE ( 'NONE', #4606, 4.000000000000000000 ) ;
#16326=AXIS2_PLACEMENT_3D ( 'NONE', #22054, #10027, #16059 ) ;
#16338=ORIENTED_EDGE ( 'NONE', *, *, #23410, .T. ) ;
#16341=PRODUCT_DEFINITION_SHAPE ( 'NONE', 'NONE',  #24993 ) ;
#16345=CARTESIAN_POINT ( 'NONE',  ( -3.756430356249996105, 26.41562499938548925, 11.16877607737301226 ) ) ;
#16349=CARTESIAN_POINT ( 'NONE',  ( -5.706339097770935176, 31.50000000000000000, 7.145898033750358813 ) ) ;
#16359=CARTESIAN_POINT ( 'NONE',  ( 3.469446951953614189E-15, 25.00000000000000000, 8.999999999999992895 ) ) ;
#16376=ORIENTED_EDGE ( 'NONE', *, *, #17841, .T. ) ;
#16403=CARTESIAN_POINT ( 'NONE',  ( 3.756430356250006319, 27.99062499938548854, 6.831223922626973533 ) ) ;
#16437=CARTESIAN_POINT ( 'NONE',  ( 8.012344526598182026E-15, 28.51562499938548356, 4.662447845253954171 ) ) ;
#16446=CARTESIAN_POINT ( 'NONE',  ( -3.756430356249996105, 28.47812499938548569, 6.831223922626973533 ) ) ;
#16448=ADVANCED_FACE ( 'NONE', ( #631 ), #8598, .F. ) ;
#16452=DIRECTION ( 'NONE',  ( 0.000000000000000000, 0.000000000000000000, 1.000000000000000000 ) ) ;
#16480=CARTESIAN_POINT ( 'NONE',  ( -1.878215178124996498, 25.85312499938548925, 5.746835883940462963 ) ) ;
#16486=CARTESIAN_POINT ( 'NONE',  ( 3.959305671612554781E-15, 35.50000000000000711, 12.99999999999999289 ) ) ;
#16498=CARTESIAN_POINT ( 'NONE',  ( 1.071796769724494114, 27.55134618820330061, 12.99999999999999112 ) ) ;
#16522=CARTESIAN_POINT ( 'NONE',  ( -1.394453263437886604E-15, 27.30624999877096926, 4.999999999999991118 ) ) ;
#16526=VERTEX_POINT ( 'NONE', #10673 ) ;
#16528=CARTESIAN_POINT ( 'NONE',  ( -3.756430356249994329, 28.59062499938548996, 6.831223922626973533 ) ) ;
#16533=VERTEX_POINT ( 'NONE', #16968 ) ;
#16540=CARTESIAN_POINT ( 'NONE',  ( 3.878215178125001827, 25.07031249969274711, 8.999999999999992895 ) ) ;
#16550=CARTESIAN_POINT ( 'NONE',  ( 4.000000000000001776, 25.84374999877097423, 8.999999999999992895 ) ) ;
#16557=CARTESIAN_POINT ( 'NONE',  ( -3.756430356249996549, 26.41562499938548925, 11.16877607737301048 ) ) ;
#16561=CARTESIAN_POINT ( 'NONE',  ( 1.071796769724495446, 27.34240381056767433, 4.999999999999992895 ) ) ;
#16562=ORIENTED_EDGE ( 'NONE', *, *, #16611, .T. ) ;
#16564=CARTESIAN_POINT ( 'NONE',  ( -1.878215178124998275, 28.59062499938548640, 12.25316411605951927 ) ) ;
#16584=ORIENTED_EDGE ( 'NONE', *, *, #3402, .T. ) ;
#16610=DIRECTION ( 'NONE',  ( 0.000000000000000000, -1.000000000000000000, 0.000000000000000000 ) ) ;
#16611=EDGE_CURVE ( 'NONE', #18643, #25109, #12657, .T. ) ;
#16625=DIRECTION ( 'NONE',  ( -0.000000000000000000, -1.000000000000000000, -0.000000000000000000 ) ) ;
#16637=CARTESIAN_POINT ( 'NONE',  ( 6.938893903907228378E-15, 31.50000000000000000, 3.499999999999992450 ) ) ;
#16643=DIRECTION ( 'NONE',  ( -0.000000000000000000, -1.000000000000000000, -0.000000000000000000 ) ) ;
#16646=CARTESIAN_POINT ( 'NONE',  ( -1.878215178124998275, 28.10312499938548925, 5.746835883940462963 ) ) ;
#16647=VERTEX_POINT ( 'NONE', #13045 ) ;
#16652=CARTESIAN_POINT ( 'NONE',  ( 3.959305671612554781E-15, 35.50000000000000711, 12.99999999999999289 ) ) ;
#16654=EDGE_LOOP ( 'NONE', ( #20667, #18419, #15463, #24721 ) ) ;
#16670=CARTESIAN_POINT ( 'NONE',  ( -3.999999999999999556, 26.10624999877097352, 11.30940107675849404 ) ) ;
#16671=CARTESIAN_POINT ( 'NONE',  ( 3.469446951953614189E-15, 31.50000000000000000, 4.999999999999992006 ) ) ;
#16674=CARTESIAN_POINT ( 'NONE',  ( 5.244320908822881933, 38.86762122992235646, 11.05479723877108178 ) ) ;
#16688=CARTESIAN_POINT ( 'NONE',  ( -3.756430356249996549, 25.36562499938548854, 8.999999999999992895 ) ) ;
#16692=CARTESIAN_POINT ( 'NONE',  ( -3.756430356249996105, 26.22812499938548569, 6.831223922626973533 ) ) ;
#16722=ORIENTED_EDGE ( 'NONE', *, *, #19586, .T. ) ;
#16725=CARTESIAN_POINT ( 'NONE',  ( 1.878215178125001605, 27.42812499938548854, 12.25316411605952283 ) ) ;
#16727=AXIS2_PLACEMENT_3D ( 'NONE', #7320, #9024, #15300 ) ;
#16737=DIRECTION ( 'NONE',  ( 0.000000000000000000, -1.000000000000000000, 0.000000000000000000 ) ) ;
#16751=LINE ( 'NONE', #2488, #23378 ) ;
#16755=EDGE_CURVE ( 'NONE', #7506, #7412, #6943, .T. ) ;
#16757=VERTEX_POINT ( 'NONE', #3994 ) ;
#16761=VECTOR ( 'NONE', #2561, 1000.000000000000000 ) ;
#16787=CARTESIAN_POINT ( 'NONE',  ( -3.756430356249994329, 29.11562499938548498, 11.16877607737301226 ) ) ;
#16791=ORIENTED_EDGE ( 'NONE', *, *, #18426, .T. ) ;
#16792=LINE ( 'NONE', #20704, #8374 ) ;
#16806=CARTESIAN_POINT ( 'NONE',  ( -3.999999999999999112, 26.61250000000000426, 11.30940107675849404 ) ) ;
#16824=CARTESIAN_POINT ( 'NONE',  ( -3.918623196469518177, 38.49999999999999289, 4.456389954662586028 ) ) ;
#16826=EDGE_CURVE ( 'NONE', #5382, #20504, #8443, .T. ) ;
#16831=CARTESIAN_POINT ( 'NONE',  ( 1.878215178125003382, 25.66562499938548214, 5.746835883940462963 ) ) ;
#16834=CARTESIAN_POINT ( 'NONE',  ( -1.859271017917182139E-15, 26.46249999999999858, 4.999999999999991118 ) ) ;
#16835=CARTESIAN_POINT ( 'NONE',  ( 0.000000000000000000, 25.78750000000000497, 13.61880215351699874 ) ) ;
#16853=CARTESIAN_POINT ( 'NONE',  ( 3.959305671612554781E-15, 35.50000000000000711, 12.99999999999999289 ) ) ;
#16855=CARTESIAN_POINT ( 'NONE',  ( 3.469446951953614189E-15, 35.50000000000000711, 8.999999999999992895 ) ) ;
#16865=ORIENTED_EDGE ( 'NONE', *, *, #17402, .F. ) ;
#16867=CARTESIAN_POINT ( 'NONE',  ( -3.756430356249996105, 27.69062499938548427, 6.831223922626973533 ) ) ;
#16898=STYLED_ITEM ( 'NONE', ( #25468 ), #4445 ) ;
#16900=CYLINDRICAL_SURFACE ( 'NONE', #24461, 4.000000000000000000 ) ;
#16912=CYLINDRICAL_SURFACE ( 'NONE', #8011, 0.5000000000000004441 ) ;
#16924=CARTESIAN_POINT ( 'NONE',  ( -1.999999999999996669, 27.94374999877097565, 12.46410161513774639 ) ) ;
#16926=DIRECTION ( 'NONE',  ( 0.000000000000000000, -1.000000000000000000, 0.000000000000000000 ) ) ;
#16938=CARTESIAN_POINT ( 'NONE',  ( -2.003086131649545506E-15, 27.08124999877097139, 13.61880215351699874 ) ) ;
#16944=CARTESIAN_POINT ( 'NONE',  ( 0.000000000000000000, 28.74062499938548854, 13.33755215474603162 ) ) ;
#16956=DIRECTION ( 'NONE',  ( -0.000000000000000000, -1.000000000000000000, -0.000000000000000000 ) ) ;
#16957=CARTESIAN_POINT ( 'NONE',  ( 4.000000000000002665, 25.48750000000000426, 6.690598923241489970 ) ) ;
#16968=CARTESIAN_POINT ( 'NONE',  ( 1.394453263437886604E-15, 28.88124999877097210, 12.99999999999999289 ) ) ;
#16978=ORIENTED_EDGE ( 'NONE', *, *, #2480, .T. ) ;
#16984=ORIENTED_EDGE ( 'NONE', *, *, #23440, .F. ) ;
#16986=CARTESIAN_POINT ( 'NONE',  ( -3.756430356249998326, 27.24062499938548854, 6.831223922626973533 ) ) ;
#16989=( NAMED_UNIT ( * ) PLANE_ANGLE_UNIT ( ) SI_UNIT ( $, .RADIAN. ) );
#17017=CARTESIAN_POINT ( 'NONE',  ( -3.110308778861272216, 31.50000000000000000, 14.13088484572967296 ) ) ;
#17019=ORIENTED_EDGE ( 'NONE', *, *, #19586, .F. ) ;
#17030=CARTESIAN_POINT ( 'NONE',  ( -8.366719580627318441E-15, 29.55624999877097281, 4.999999999999992006 ) ) ;
#17035=VERTEX_POINT ( 'NONE', #18455 ) ;
#17037=FACE_OUTER_BOUND ( 'NONE', #15236, .T. ) ;
#17052=DIRECTION ( 'NONE',  ( -0.000000000000000000, -1.000000000000000000, -0.000000000000000000 ) ) ;
#17054=VECTOR ( 'NONE', #18442, 1000.000000000000114 ) ;
#17059=CARTESIAN_POINT ( 'NONE',  ( 0.000000000000000000, 28.43124999877097636, 13.61880215351699874 ) ) ;
#17072=VECTOR ( 'NONE', #13077, 1000.000000000000000 ) ;
#17078=CARTESIAN_POINT ( 'NONE',  ( 3.756430356250003211, 29.19062499938548072, 8.999999999999992895 ) ) ;
#17081=DIRECTION ( 'NONE',  ( 0.000000000000000000, 0.000000000000000000, 1.000000000000000000 ) ) ;
#17087=AXIS2_PLACEMENT_3D ( 'NONE', #17388, #25485, #5347 ) ;
#17088=CARTESIAN_POINT ( 'NONE',  ( -1.071796769724487675, 26.87634618820331411, 4.999999999999992895 ) ) ;
#17110=CARTESIAN_POINT ( 'NONE',  ( 3.756430356250000546, 28.36562499938549564, 11.16877607737301226 ) ) ;
#17121=CARTESIAN_POINT ( 'NONE',  ( 4.000000000000007105, 29.08750000000000568, 6.690598923241489970 ) ) ;
#17135=CYLINDRICAL_SURFACE ( 'NONE', #10550, 0.5000000000000004441 ) ;
#17143=ORIENTED_EDGE ( 'NONE', *, *, #22508, .F. ) ;
#17164=CARTESIAN_POINT ( 'NONE',  ( -1.999999999999994893, 29.59374999877097068, 5.535898384862237620 ) ) ;
#17177=ORIENTED_EDGE ( 'NONE', *, *, #25793, .T. ) ;
#17201=CARTESIAN_POINT ( 'NONE',  ( 4.000000000000003553, 26.74374999877097281, 8.999999999999992895 ) ) ;
#17209=VERTEX_POINT ( 'NONE', #21063 ) ;
#17217=CARTESIAN_POINT ( 'NONE',  ( -3.756430356249996549, 26.22812499938548569, 6.831223922626973533 ) ) ;
#17218=CIRCLE ( 'NONE', #12612, 0.5000000000000004441 ) ;
#17219=CARTESIAN_POINT ( 'NONE',  ( 6.009258394948636914E-15, 29.30312499938549564, 4.662447845253954171 ) ) ;
#17220=CIRCLE ( 'NONE', #23459, 6.000000000000000000 ) ;
#17250=EDGE_LOOP ( 'NONE', ( #7230, #5653, #6218, #11081 ) ) ;
#17251=ORIENTED_EDGE ( 'NONE', *, *, #9867, .F. ) ;
#17252=DIRECTION ( 'NONE',  ( 0.000000000000000000, 0.000000000000000000, 1.000000000000000000 ) ) ;
#17253=CARTESIAN_POINT ( 'NONE',  ( -1.878215178124998275, 28.25312499938548783, 12.25316411605951927 ) ) ;
#17275=VERTEX_POINT ( 'NONE', #21312 ) ;
#17276=CARTESIAN_POINT ( 'NONE',  ( 3.756430356250003211, 29.30312499938548498, 8.999999999999992895 ) ) ;
#17283=VERTEX_POINT ( 'NONE', #25108 ) ;
#17287=CARTESIAN_POINT ( 'NONE',  ( 3.756430356250006319, 25.17812499938548854, 6.831223922626973533 ) ) ;
#17296=FACE_OUTER_BOUND ( 'NONE', #14888, .T. ) ;
#17320=CARTESIAN_POINT ( 'NONE',  ( -3.999999999999996447, 25.63750000000000284, 6.690598923241487306 ) ) ;
#17329=CARTESIAN_POINT ( 'NONE',  ( -1.999999999999994893, 28.24374999877096926, 5.535898384862237620 ) ) ;
#17334=DIRECTION ( 'NONE',  ( 0.000000000000000000, 1.000000000000000000, 0.000000000000000000 ) ) ;
#17337=ORIENTED_EDGE ( 'NONE', *, *, #9365, .T. ) ;
#17344=CARTESIAN_POINT ( 'NONE',  ( -3.756430356249994773, 28.06562499938548783, 8.999999999999992895 ) ) ;
#17347=CARTESIAN_POINT ( 'NONE',  ( 4.000000000000005329, 25.03750000000000142, 6.690598923241489970 ) ) ;
#17364=CARTESIAN_POINT ( 'NONE',  ( 8.012344526598182026E-15, 25.81562499938549138, 4.662447845253954171 ) ) ;
#17367=CARTESIAN_POINT ( 'NONE',  ( 6.972266317189432034E-15, 28.65624999877097423, 4.999999999999992006 ) ) ;
#17372=CARTESIAN_POINT ( 'NONE',  ( 3.756430356250004543, 29.34062499938548640, 6.831223922626973533 ) ) ;
#17388=CARTESIAN_POINT ( 'NONE',  ( -3.526711513754876570, 29.50000000000000000, 4.145898033750337497 ) ) ;
#17402=EDGE_CURVE ( 'NONE', #15841, #32, #21985, .T. ) ;
#17403=CARTESIAN_POINT ( 'NONE',  ( 1.878215178124998275, 25.51562499938548711, 12.25316411605952283 ) ) ;
#17424=ORIENTED_EDGE ( 'NONE', *, *, #12141, .F. ) ;
#17425=DIRECTION ( 'NONE',  ( -0.000000000000000000, 1.000000000000000000, -0.000000000000000000 ) ) ;
#17443=CARTESIAN_POINT ( 'NONE',  ( 4.000000000000000888, 28.95624999877097494, 11.30940107675849760 ) ) ;
#17454=CARTESIAN_POINT ( 'NONE',  ( 3.289814793420742678, 38.99786504297400569, 4.589397325852536014 ) ) ;
#17456=CARTESIAN_POINT ( 'NONE',  ( -3.756430356249996549, 27.12812499938548783, 6.831223922626973533 ) ) ;
#17458=CARTESIAN_POINT ( 'NONE',  ( 4.000000000000001776, 26.35000000000000497, 8.999999999999992895 ) ) ;
#17471=( BOUNDED_CURVE ( )  B_SPLINE_CURVE ( 2, ( #11676, #3966, #7634, #13646, #10103, #13527, #1613, #23703, #8152 ),
 .UNSPECIFIED., .F., .F. ) 
 B_SPLINE_CURVE_WITH_KNOTS ( ( 3, 2, 2, 2, 3 ),
 ( 0.6750000000000000444, 0.6833333333333333481, 0.6999999999999999556, 0.7166666666666666741, 0.7249999999999999778 ),
 .UNSPECIFIED. ) 
 CURVE ( )  GEOMETRIC_REPRESENTATION_ITEM ( )  RATIONAL_B_SPLINE_CURVE ( ( 0.9330127018922194093, 0.9330127018922198534, 1.000000000000000000, 0.8660254037844387076, 1.000000000000000000, 0.8660254037844387076, 1.000000000000000000, 0.9330127018922194093, 0.9330127018922194093 ) ) 
 REPRESENTATION_ITEM ( '' )  );
#17475=DIRECTION ( 'NONE',  ( -0.000000000000000000, -1.000000000000000000, -0.000000000000000000 ) ) ;
#17487=CARTESIAN_POINT ( 'NONE',  ( -3.756430356249998326, 25.85312499938549635, 11.16877607737301226 ) ) ;
#17501=ORIENTED_EDGE ( 'NONE', *, *, #10900, .F. ) ;
#17505=ADVANCED_FACE ( 'NONE', ( #4160 ), #4687, .F. ) ;
#17508=CARTESIAN_POINT ( 'NONE',  ( 4.648177544792955347E-16, 28.93750000000000355, 12.99999999999999289 ) ) ;
#17511=CARTESIAN_POINT ( 'NONE',  ( -3.756430356250000546, 29.56562499938549493, 11.16877607737301226 ) ) ;
#17512=CARTESIAN_POINT ( 'NONE',  ( -5.218519194534875894, 39.00427158776031433, 7.275297520595652045 ) ) ;
#17520=ORIENTED_EDGE ( 'NONE', *, *, #5020, .T. ) ;
#17524=EDGE_CURVE ( 'NONE', #6543, #9952, #12496, .T. ) ;
#17535=DIRECTION ( 'NONE',  ( 0.000000000000000000, -1.000000000000000000, -0.000000000000000000 ) ) ;
#17540=LINE ( 'NONE', #1191, #5360 ) ;
#17552=ORIENTED_EDGE ( 'NONE', *, *, #18420, .T. ) ;
#17567=AXIS2_PLACEMENT_3D ( 'NONE', #6529, #17919, #10 ) ;
#17574=VERTEX_POINT ( 'NONE', #4301 ) ;
#17576=CARTESIAN_POINT ( 'NONE',  ( -2.003086131649545506E-15, 29.78124999877097778, 13.61880215351699874 ) ) ;
#17591=CARTESIAN_POINT ( 'NONE',  ( -1.878215178124996498, 28.89062499938548711, 5.746835883940462963 ) ) ;
#17592=CARTESIAN_POINT ( 'NONE',  ( 0.4553717634079643695, 38.72245023127408814, 3.239938118008596213 ) ) ;
#17593=CARTESIAN_POINT ( 'NONE',  ( 2.003086131649545506E-15, 27.58750000000000568, 13.61880215351699874 ) ) ;
#17595=FACE_OUTER_BOUND ( 'NONE', #23329, .T. ) ;
#17603=CIRCLE ( 'NONE', #10914, 5.000000000000000888 ) ;
#17611=CARTESIAN_POINT ( 'NONE',  ( -3.756430356249996549, 25.89062499938548356, 6.831223922626973533 ) ) ;
#17624=CARTESIAN_POINT ( 'NONE',  ( -3.756430356249994329, 29.11562499938548498, 11.16877607737301226 ) ) ;
#17625=VECTOR ( 'NONE', #15320, 1000.000000000000000 ) ;
#17630=DIRECTION ( 'NONE',  ( 0.000000000000000000, 1.000000000000000000, 0.000000000000000000 ) ) ;
#17632=FACE_OUTER_BOUND ( 'NONE', #17776, .T. ) ;
#17641=VERTEX_POINT ( 'NONE', #20239 ) ;
#17649=DIRECTION ( 'NONE',  ( 0.000000000000000000, -0.000000000000000000, 1.000000000000000000 ) ) ;
#17673=DIRECTION ( 'NONE',  ( 0.000000000000000000, 0.000000000000000000, 1.000000000000000000 ) ) ;
#17686=CARTESIAN_POINT ( 'NONE',  ( -1.999999999999998224, 26.95000000000000639, 5.535898384862237620 ) ) ;
#17696=ORIENTED_EDGE ( 'NONE', *, *, #11851, .T. ) ;
#17700=( GEOMETRIC_REPRESENTATION_CONTEXT ( 3 ) GLOBAL_UNCERTAINTY_ASSIGNED_CONTEXT ( ( #25095 ) ) GLOBAL_UNIT_ASSIGNED_CONTEXT ( ( #6131, #23928, #19743 ) ) REPRESENTATION_CONTEXT ( 'NONE', 'WORKASPACE' ) );
#17702=CARTESIAN_POINT ( 'NONE',  ( -1.071796769724485232, 25.58259618943233704, 4.999999999999992006 ) ) ;
#17712=CARTESIAN_POINT ( 'NONE',  ( -3.999999999999994671, 29.70624999877097494, 11.30940107675849404 ) ) ;
#17714=CARTESIAN_POINT ( 'NONE',  ( -1.999999999999994893, 29.20000000000000284, 5.535898384862237620 ) ) ;
#17719=ORIENTED_EDGE ( 'NONE', *, *, #12171, .T. ) ;
#17720=CARTESIAN_POINT ( 'NONE',  ( 3.338448572212769694, 38.98643850599027161, 4.611800620969658482 ) ) ;
#17723=CARTESIAN_POINT ( 'NONE',  ( 1.878215178125001605, 27.31562499938548783, 12.25316411605952283 ) ) ;
#17725=CARTESIAN_POINT ( 'NONE',  ( 2.000000000000000000, 27.17500000000000426, 12.46410161513774817 ) ) ;
#17742=CARTESIAN_POINT ( 'NONE',  ( 3.756430356250002323, 26.11562499938549564, 11.16877607737301403 ) ) ;
#17749=FACE_OUTER_BOUND ( 'NONE', #18107, .T. ) ;
#17750=CARTESIAN_POINT ( 'NONE',  ( 3.756430356250004543, 26.00312499938548783, 11.16877607737301226 ) ) ;
#17765=CARTESIAN_POINT ( 'NONE',  ( -5.306793332224213344, 38.77026726007181878, 11.16082596406551986 ) ) ;
#17766=CARTESIAN_POINT ( 'NONE',  ( 5.239883324427840883, 38.87578012723909637, 6.956022275050601777 ) ) ;
#17776=EDGE_LOOP ( 'NONE', ( #8764, #24858, #11109, #9287 ) ) ;
#17780=AXIS2_PLACEMENT_3D ( 'NONE', #6161, #16625, #22896 ) ;
#17781=EDGE_LOOP ( 'NONE', ( #3424, #13344, #21207, #16722 ) ) ;
#17787=CARTESIAN_POINT ( 'NONE',  ( -2.003086131649545506E-15, 26.37812499938548427, 13.33755215474602984 ) ) ;
#17793=EDGE_CURVE ( 'NONE', #13062, #1533, #21032, .T. ) ;
#17795=CARTESIAN_POINT ( 'NONE',  ( -0.4995657836784060390, 31.50000000000000000, 14.97916666666665897 ) ) ;
#17798=CARTESIAN_POINT ( 'NONE',  ( 4.000000000000002665, 26.33124999877097494, 6.690598923241489970 ) ) ;
#17832=CARTESIAN_POINT ( 'NONE',  ( 3.756430356250002323, 26.11562499938549564, 11.16877607737301226 ) ) ;
#17841=EDGE_CURVE ( 'NONE', #17283, #24856, #23497, .T. ) ;
#17843=CARTESIAN_POINT ( 'NONE',  ( -3.999999999999999112, 26.03124999877097423, 6.690598923241487306 ) ) ;
#17847=CARTESIAN_POINT ( 'NONE',  ( 3.756430356250003211, 29.19062499938548072, 8.999999999999992895 ) ) ;
#17849=CARTESIAN_POINT ( 'NONE',  ( -1.999999999999998224, 28.00000000000000711, 12.46410161513774639 ) ) ;
#17863=DIRECTION ( 'NONE',  ( 0.000000000000000000, 1.000000000000000000, 0.000000000000000000 ) ) ;
#17867=CARTESIAN_POINT ( 'NONE',  ( -1.878215178124996498, 25.85312499938548925, 5.746835883940462963 ) ) ;
#17872=CARTESIAN_POINT ( 'NONE',  ( 1.859271017917182139E-15, 29.38750000000000639, 12.99999999999999289 ) ) ;
#17876=CARTESIAN_POINT ( 'NONE',  ( 3.756430356250004987, 26.49062499938548854, 8.999999999999992895 ) ) ;
#17880=CARTESIAN_POINT ( 'NONE',  ( -0.4995657836784084815, 38.49999999999999289, 14.97916666666665897 ) ) ;
#17886=DIRECTION ( 'NONE',  ( 0.000000000000000000, 0.000000000000000000, 1.000000000000000000 ) ) ;
#17893=CARTESIAN_POINT ( 'NONE',  ( 3.034965225792634058, 38.86762122992235646, 13.74490037465567127 ) ) ;
#17896=CARTESIAN_POINT ( 'NONE',  ( -5.207925457499139377, 38.94727318402490113, 7.073160566612318512 ) ) ;
#17901=EDGE_CURVE ( 'NONE', #5382, #2175, #20292, .T. ) ;
#17907=CIRCLE ( 'NONE', #14979, 6.000000000000000000 ) ;
#17909=CARTESIAN_POINT ( 'NONE',  ( -1.878215178124999829, 26.34062499938548996, 12.25316411605951927 ) ) ;
#17919=DIRECTION ( 'NONE',  ( -0.000000000000000000, -1.000000000000000000, -0.000000000000000000 ) ) ;
#17933=( BOUNDED_CURVE ( )  B_SPLINE_CURVE ( 2, ( #6117, #25869, #20107, #21685, #247, #21826, #25738, #8216, #12130 ),
 .UNSPECIFIED., .F., .F. ) 
 B_SPLINE_CURVE_WITH_KNOTS ( ( 3, 2, 2, 2, 3 ),
 ( 0.8250000000000000666, 0.8333333333333333703, 0.8499999999999999778, 0.8666666666666666963, 0.8750000000000000000 ),
 .UNSPECIFIED. ) 
 CURVE ( )  GEOMETRIC_REPRESENTATION_ITEM ( )  RATIONAL_B_SPLINE_CURVE ( ( 0.9330127018922194093, 0.9330127018922198534, 1.000000000000000000, 0.8660254037844387076, 1.000000000000000000, 0.8660254037844387076, 1.000000000000000000, 0.9330127018922194093, 0.9330127018922194093 ) ) 
 REPRESENTATION_ITEM ( '' )  );
#17965=CARTESIAN_POINT ( 'NONE',  ( 8.012344526598182026E-15, 25.81562499938549138, 4.662447845253954171 ) ) ;
#17977=CARTESIAN_POINT ( 'NONE',  ( 0.07793552093708305817, 39.00000000000049027, 14.49999999999953992 ) ) ;
#17983=CARTESIAN_POINT ( 'NONE',  ( -1.999999999999998224, 26.65000000000000568, 12.46410161513774639 ) ) ;
#18003=CARTESIAN_POINT ( 'NONE',  ( 4.006172263299091013E-15, 26.71562499938548640, 4.662447845253954171 ) ) ;
#18013=CARTESIAN_POINT ( 'NONE',  ( -3.756430356249996549, 27.61562499938548143, 8.999999999999992895 ) ) ;
#18032=CARTESIAN_POINT ( 'NONE',  ( -5.297276937894413784, 38.97868814324866804, 10.55807547785406797 ) ) ;
#18033=CARTESIAN_POINT ( 'NONE',  ( 5.357761973269630218, 38.93893882358702285, 7.509353182747807054 ) ) ;
#18038=LINE ( 'NONE', #123, #23758 ) ;
#18039=CARTESIAN_POINT ( 'NONE',  ( 3.843461816822868027, 38.61000136877623135, 13.46319918748939948 ) ) ;
#18041=CARTESIAN_POINT ( 'NONE',  ( 7.437084071668728555E-15, 26.63124999877097565, 12.99999999999999112 ) ) ;
#18049=ORIENTED_EDGE ( 'NONE', *, *, #15099, .F. ) ;
#18055=CARTESIAN_POINT ( 'NONE',  ( 3.756430356250002323, 27.80312499938548854, 11.16877607737301226 ) ) ;
#18067=CARTESIAN_POINT ( 'NONE',  ( 9.296355089585910693E-16, 26.18124999877096926, 12.99999999999999289 ) ) ;
#18073=EDGE_CURVE ( 'NONE', #1503, #8259, #17540, .T. ) ;
#18074=CARTESIAN_POINT ( 'NONE',  ( 2.000000000000005329, 28.16874999877097352, 5.535898384862238508 ) ) ;
#18077=CARTESIAN_POINT ( 'NONE',  ( -1.999999999999998224, 27.10000000000000497, 12.46410161513774639 ) ) ;
#18083=ORIENTED_EDGE ( 'NONE', *, *, #4824, .T. ) ;
#18096=CARTESIAN_POINT ( 'NONE',  ( 3.469446951953614189E-15, 35.50000000000000711, 8.999999999999992895 ) ) ;
#18101=FACE_OUTER_BOUND ( 'NONE', #8105, .T. ) ;
#18107=EDGE_LOOP ( 'NONE', ( #22608, #25459, #18798, #23303 ) ) ;
#18108=CARTESIAN_POINT ( 'NONE',  ( 3.756430356250003211, 26.15312499938548996, 8.999999999999992895 ) ) ;
#18114=CARTESIAN_POINT ( 'NONE',  ( -1.071796769724492782, 29.18259618943233491, 4.999999999999995559 ) ) ;
#18143=CARTESIAN_POINT ( 'NONE',  ( -1.878215178124999829, 26.45312499938549422, 12.25316411605951927 ) ) ;
#18151=CARTESIAN_POINT ( 'NONE',  ( -5.706339097770935176, 31.50000000000000000, 7.145898033750358813 ) ) ;
#18152=CARTESIAN_POINT ( 'NONE',  ( -3.756430356249998326, 28.02812499938548640, 6.831223922626973533 ) ) ;
#18182=CARTESIAN_POINT ( 'NONE',  ( -3.756430356249998326, 28.02812499938548640, 6.831223922626973533 ) ) ;
#18204=ORIENTED_EDGE ( 'NONE', *, *, #24600, .T. ) ;
#18225=CARTESIAN_POINT ( 'NONE',  ( 4.006172263299091013E-15, 27.16562499938548569, 4.662447845253954171 ) ) ;
#18233=EDGE_CURVE ( 'NONE', #1729, #14559, #2421, .T. ) ;
#18250=ORIENTED_EDGE ( 'NONE', *, *, #113, .T. ) ;
#18253=CARTESIAN_POINT ( 'NONE',  ( -3.756430356249997882, 28.14062499938548356, 6.831223922626973533 ) ) ;
#18257=CARTESIAN_POINT ( 'NONE',  ( 4.000000000000005329, 27.25000000000000355, 8.999999999999992895 ) ) ;
#18260=ORIENTED_EDGE ( 'NONE', *, *, #2082, .F. ) ;
#18262=CARTESIAN_POINT ( 'NONE',  ( -3.756430356249996105, 27.12812499938548783, 6.831223922626973533 ) ) ;
#18265=CARTESIAN_POINT ( 'NONE',  ( 4.000000000000005329, 26.38750000000000995, 6.690598923241489970 ) ) ;
#18269=DIRECTION ( 'NONE',  ( 0.000000000000000000, 1.000000000000000000, 0.000000000000000000 ) ) ;
#18292=ORIENTED_EDGE ( 'NONE', *, *, #22216, .T. ) ;
#18298=CARTESIAN_POINT ( 'NONE',  ( 5.112995299272250684E-15, 27.75624999877097565, 4.999999999999992006 ) ) ;
#18309=EDGE_CURVE ( 'NONE', #9952, #6478, #20802, .T. ) ;
#18315=ORIENTED_EDGE ( 'NONE', *, *, #6789, .F. ) ;
#18316=CARTESIAN_POINT ( 'NONE',  ( 1.071796769724495446, 27.73615380933864571, 4.999999999999992895 ) ) ;
#18319=ORIENTED_EDGE ( 'NONE', *, *, #12503, .F. ) ;
#18320=ORIENTED_EDGE ( 'NONE', *, *, #2801, .F. ) ;
#18347=CARTESIAN_POINT ( 'NONE',  ( -3.756430356249998326, 28.14062499938548356, 6.831223922626973533 ) ) ;
#18351=DIRECTION ( 'NONE',  ( -0.000000000000000000, -1.000000000000000000, -0.000000000000000000 ) ) ;
#18363=CARTESIAN_POINT ( 'NONE',  ( 2.003086131649545506E-15, 29.38750000000000284, 13.61880215351699874 ) ) ;
#18370=CARTESIAN_POINT ( 'NONE',  ( -0.4451413195715977489, 38.71736240459208034, 3.234498339501550745 ) ) ;
#18374=CARTESIAN_POINT ( 'NONE',  ( 5.396012270207167560, 38.91143067427094593, 10.45569860586814137 ) ) ;
#18379=CARTESIAN_POINT ( 'NONE',  ( 1.878215178125005158, 28.47812499938549280, 5.746835883940462963 ) ) ;
#18390=CARTESIAN_POINT ( 'NONE',  ( -1.878215178124996498, 27.54062499938548569, 5.746835883940462963 ) ) ;
#18410=EDGE_LOOP ( 'NONE', ( #12554, #10330, #18250, #21450 ) ) ;
#18414=EDGE_LOOP ( 'NONE', ( #9058, #13476, #22342, #16018 ) ) ;
#18416=DIRECTION ( 'NONE',  ( 0.000000000000000000, 1.000000000000000000, 0.000000000000000000 ) ) ;
#18419=ORIENTED_EDGE ( 'NONE', *, *, #1174, .T. ) ;
#18420=EDGE_CURVE ( 'NONE', #17283, #18643, #9949, .T. ) ;
#18426=EDGE_CURVE ( 'NONE', #19882, #5382, #12412, .T. ) ;
#18430=CARTESIAN_POINT ( 'NONE',  ( -3.918623196469422698, 38.49999999999999289, 13.54361004533748059 ) ) ;
#18442=DIRECTION ( 'NONE',  ( -0.8660254037844395958, -0.4999999999999982792, 0.000000000000000000 ) ) ;
#18455=CARTESIAN_POINT ( 'NONE',  ( 5.112995299272250684E-15, 26.01250000000000284, 4.999999999999992006 ) ) ;
#18478=DIRECTION ( 'NONE',  ( -0.000000000000000000, -1.000000000000000000, -0.000000000000000000 ) ) ;
#18484=( BOUNDED_CURVE ( )  B_SPLINE_CURVE ( 2, ( #2389, #24226, #6694, #24609, #8659 ),
 .UNSPECIFIED., .F., .F. ) 
 B_SPLINE_CURVE_WITH_KNOTS ( ( 3, 2, 3 ),
 ( 0.000000000000000000, 0.01666666666666666644, 0.02500000000000000486 ),
 .UNSPECIFIED. ) 
 CURVE ( )  GEOMETRIC_REPRESENTATION_ITEM ( )  RATIONAL_B_SPLINE_CURVE ( ( 1.000000000000000000, 0.8660254037844387076, 1.000000000000000000, 0.9330127018922192983, 0.9330127018922194093 ) ) 
 REPRESENTATION_ITEM ( '' )  );
#18490=CARTESIAN_POINT ( 'NONE',  ( -1.878215178124996498, 27.20312499938549067, 5.746835883940462963 ) ) ;
#18496=CARTESIAN_POINT ( 'NONE',  ( -3.999999999999999112, 28.41250000000000497, 11.30940107675849404 ) ) ;
#18497=VERTEX_POINT ( 'NONE', #5220 ) ;
#18499=EDGE_CURVE ( 'NONE', #9321, #14559, #11098, .T. ) ;
#18505=VECTOR ( 'NONE', #19182, 1000.000000000000000 ) ;
#18514=CARTESIAN_POINT ( 'NONE',  ( -1.999999999999996669, 25.69374999877097920, 12.46410161513774639 ) ) ;
#18522=CARTESIAN_POINT ( 'NONE',  ( 3.756430356250003211, 27.05312499938548854, 8.999999999999992895 ) ) ;
#18532=CARTESIAN_POINT ( 'NONE',  ( 3.756430356250003211, 28.29062499938548569, 8.999999999999992895 ) ) ;
#18534=ADVANCED_FACE ( 'NONE', ( #10974 ), #1549, .F. ) ;
#18555=DIRECTION ( 'NONE',  ( 0.000000000000000000, 0.000000000000000000, -1.000000000000000000 ) ) ;
#18558=DIRECTION ( 'NONE',  ( 0.000000000000000000, 1.000000000000000000, 0.000000000000000000 ) ) ;
#18565=CARTESIAN_POINT ( 'NONE',  ( -1.878215178124998275, 26.00312499938549493, 12.25316411605951927 ) ) ;
#18571=CARTESIAN_POINT ( 'NONE',  ( -3.077479918315519036, 38.94082980537690020, 4.370215950314418230 ) ) ;
#18578=CARTESIAN_POINT ( 'NONE',  ( -3.999999999999999112, 27.43750000000001066, 6.690598923241487306 ) ) ;
#18583=CARTESIAN_POINT ( 'NONE',  ( 7.901901826148023498E-15, 27.53124999877097068, 12.99999999999999112 ) ) ;
#18592=DIRECTION ( 'NONE',  ( -0.000000000000000000, -1.000000000000000000, -0.000000000000000000 ) ) ;
#18607=CARTESIAN_POINT ( 'NONE',  ( -3.999999999999998224, 29.66874999877097352, 8.999999999999992895 ) ) ;
#18612=CARTESIAN_POINT ( 'NONE',  ( -1.878215178124999829, 28.70312499938548711, 12.25316411605951927 ) ) ;
#18615=ORIENTED_EDGE ( 'NONE', *, *, #24680, .F. ) ;
#18621=CARTESIAN_POINT ( 'NONE',  ( -0.07783014623660702846, 38.99999999999950262, 14.50000000000044587 ) ) ;
#18642=CARTESIAN_POINT ( 'NONE',  ( 4.006172263299091013E-15, 28.96562499938549351, 4.662447845253954171 ) ) ;
#18643=VERTEX_POINT ( 'NONE', #21677 ) ;
#18651=CARTESIAN_POINT ( 'NONE',  ( -1.878215178124998275, 26.79062499938548569, 12.25316411605951927 ) ) ;
#18653=CARTESIAN_POINT ( 'NONE',  ( 5.840899737312971851, 31.50000000000000000, 7.627451181685208859 ) ) ;
#18673=CARTESIAN_POINT ( 'NONE',  ( 4.000000000000000888, 29.85624999877096997, 11.30940107675849760 ) ) ;
#18677=VERTEX_POINT ( 'NONE', #2063 ) ;
#18698=VERTEX_POINT ( 'NONE', #115 ) ;
#18707=ORIENTED_EDGE ( 'NONE', *, *, #19537, .T. ) ;
#18708=CARTESIAN_POINT ( 'NONE',  ( 5.840899737312971851, 38.49999999999999289, 7.627451181685208859 ) ) ;
#18717=EDGE_CURVE ( 'NONE', #10619, #18643, #17907, .T. ) ;
#18718=LINE ( 'NONE', #5132, #5021 ) ;
#18721=CARTESIAN_POINT ( 'NONE',  ( -1.999999999999996669, 29.74374999877097636, 12.46410161513774639 ) ) ;
#18729=CARTESIAN_POINT ( 'NONE',  ( 3.756430356250001434, 27.50312499938548783, 8.999999999999992895 ) ) ;
#18732=DIRECTION ( 'NONE',  ( -0.000000000000000000, -1.000000000000000000, -0.000000000000000000 ) ) ;
#18755=CARTESIAN_POINT ( 'NONE',  ( -1.999999999999994893, 26.44374999877097210, 5.535898384862237620 ) ) ;
#18772=CARTESIAN_POINT ( 'NONE',  ( 6.009258394948636914E-15, 29.30312499938549564, 4.662447845253954171 ) ) ;
#18774=CARTESIAN_POINT ( 'NONE',  ( -3.756430356249996549, 25.40312499938548640, 11.16877607737301048 ) ) ;
#18776=EDGE_CURVE ( 'NONE', #11111, #22395, #4371, .T. ) ;
#18777=CARTESIAN_POINT ( 'NONE',  ( 2.000000000000000000, 26.27500000000000568, 12.46410161513774817 ) ) ;
#18778=CARTESIAN_POINT ( 'NONE',  ( -4.000000000000000888, 25.71250000000000568, 11.30940107675849404 ) ) ;
#18798=ORIENTED_EDGE ( 'NONE', *, *, #9343, .T. ) ;
#18799=CARTESIAN_POINT ( 'NONE',  ( -5.840899737312954976, 31.50000000000000000, 10.37254881831481690 ) ) ;
#18807=ADVANCED_FACE ( 'NONE', ( #22416 ), #24508, .F. ) ;
#18812=CARTESIAN_POINT ( 'NONE',  ( -1.878215178124998275, 28.10312499938548925, 5.746835883940462963 ) ) ;
#18817=AXIS2_PLACEMENT_3D ( 'NONE', #21407, #17475, #19815 ) ;
#18819=CARTESIAN_POINT ( 'NONE',  ( -3.290218409505503150, 38.99776139129450314, 4.589573109331187339 ) ) ;
#18821=AXIS2_PLACEMENT_3D ( 'NONE', #21746, #13766, #3829 ) ;
#18837=CARTESIAN_POINT ( 'NONE',  ( 4.000000000000003553, 27.64374999877097139, 8.999999999999992895 ) ) ;
#18839=ORIENTED_EDGE ( 'NONE', *, *, #18073, .F. ) ;
#18862=CARTESIAN_POINT ( 'NONE',  ( -5.532151103383255553, 34.50000000000000000, 6.677220593914389823 ) ) ;
#18866=CARTESIAN_POINT ( 'NONE',  ( -5.840899737312982509, 38.49999999999999289, 7.627451181685283466 ) ) ;
#18869=CARTESIAN_POINT ( 'NONE',  ( 3.718542035834364277E-15, 25.11250000000000782, 4.999999999999992006 ) ) ;
#18898=ORIENTED_EDGE ( 'NONE', *, *, #22465, .F. ) ;
#18900=CARTESIAN_POINT ( 'NONE',  ( 2.000000000000005329, 25.46874999877096712, 5.535898384862238508 ) ) ;
#18916=CARTESIAN_POINT ( 'NONE',  ( -2.000000000000000000, 25.30000000000001137, 12.46410161513774639 ) ) ;
#18918=CARTESIAN_POINT ( 'NONE',  ( 2.000000000000000000, 25.37500000000000355, 12.46410161513774817 ) ) ;
#18923=AXIS2_PLACEMENT_3D ( 'NONE', #18151, #5975, #7932 ) ;
#18947=CARTESIAN_POINT ( 'NONE',  ( -3.756430356249998326, 28.66562499938548925, 11.16877607737301226 ) ) ;
#18951=CARTESIAN_POINT ( 'NONE',  ( -3.163547630074431627, 38.99403850649169812, 4.493343988836014269 ) ) ;
#18964=AXIS2_PLACEMENT_3D ( 'NONE', #5299, #13418, #11171 ) ;
#18974=ORIENTED_EDGE ( 'NONE', *, *, #23256, .T. ) ;
#18988=CARTESIAN_POINT ( 'NONE',  ( -5.706339097770935176, 29.50000000000000000, 7.145898033750358813 ) ) ;
#18992=ADVANCED_FACE ( 'NONE', ( #13503 ), #21474, .T. ) ;
#19016=CARTESIAN_POINT ( 'NONE',  ( -1.999999999999993117, 27.34374999877097068, 5.535898384862237620 ) ) ;
#19031=CARTESIAN_POINT ( 'NONE',  ( -5.532151103383212032, 31.50000000000000000, 11.32277940608570432 ) ) ;
#19032=CARTESIAN_POINT ( 'NONE',  ( 3.756430356250000546, 25.55312499938548854, 11.16877607737301403 ) ) ;
#19035=CARTESIAN_POINT ( 'NONE',  ( 3.756430356250004543, 28.70312499938549067, 11.16877607737301226 ) ) ;
#19036=DIRECTION ( 'NONE',  ( 0.000000000000000000, 1.000000000000000000, 0.000000000000000000 ) ) ;
#19056=EDGE_CURVE ( 'NONE', #13467, #16526, #12423, .T. ) ;
#19064=CARTESIAN_POINT ( 'NONE',  ( 3.756430356250003211, 27.05312499938548854, 8.999999999999992895 ) ) ;
#19071=CARTESIAN_POINT ( 'NONE',  ( -1.022599059854450137E-14, 29.16250000000000497, 4.999999999999992006 ) ) ;
#19084=VERTEX_POINT ( 'NONE', #20140 ) ;
#19113=ORIENTED_EDGE ( 'NONE', *, *, #15329, .T. ) ;
#19134=CARTESIAN_POINT ( 'NONE',  ( 5.840899737312979845, 31.50000000000000000, 10.37254881831474052 ) ) ;
#19137=CARTESIAN_POINT ( 'NONE',  ( 0.000000000000000000, 27.53124999877097423, 13.61880215351699874 ) ) ;
#19144=ORIENTED_EDGE ( 'NONE', *, *, #11851, .F. ) ;
#19145=ORIENTED_EDGE ( 'NONE', *, *, #20794, .F. ) ;
#19152=CARTESIAN_POINT ( 'NONE',  ( 3.756430356250000546, 29.15312499938548996, 11.16877607737301226 ) ) ;
#19155=CARTESIAN_POINT ( 'NONE',  ( -4.000000000000000000, 25.67500000000000426, 8.999999999999992895 ) ) ;
#19156=ADVANCED_FACE ( 'NONE', ( #4054 ), #21721, .F. ) ;
#19178=ORIENTED_EDGE ( 'NONE', *, *, #4769, .T. ) ;
#19182=DIRECTION ( 'NONE',  ( -0.000000000000000000, 1.000000000000000000, 0.000000000000000000 ) ) ;
#19183=CARTESIAN_POINT ( 'NONE',  ( 3.756430356250004543, 27.54062499938548925, 6.831223922626973533 ) ) ;
#19198=DIRECTION ( 'NONE',  ( 0.000000000000000000, 0.000000000000000000, -1.000000000000000000 ) ) ;
#19204=FACE_OUTER_BOUND ( 'NONE', #1886, .T. ) ;
#19213=ORIENTED_EDGE ( 'NONE', *, *, #6636, .F. ) ;
#19215=VERTEX_POINT ( 'NONE', #924 ) ;
#19222=VECTOR ( 'NONE', #6828, 1000.000000000000000 ) ;
#19239=CARTESIAN_POINT ( 'NONE',  ( -1.071796769724487453, 25.31740381056767930, 12.99999999999999467 ) ) ;
#19246=VECTOR ( 'NONE', #4177, 1000.000000000000000 ) ;
#19270=CARTESIAN_POINT ( 'NONE',  ( -1.999999999999993117, 28.69374999877097210, 5.535898384862237620 ) ) ;
#19274=AXIS2_PLACEMENT_3D ( 'NONE', #25263, #10866, #5373 ) ;
#19287=CARTESIAN_POINT ( 'NONE',  ( -3.756430356249997882, 27.20312499938549067, 11.16877607737301048 ) ) ;
#19290=CARTESIAN_POINT ( 'NONE',  ( -1.878215178124996498, 28.89062499938548711, 5.746835883940462963 ) ) ;
#19303=CARTESIAN_POINT ( 'NONE',  ( -3.526711513754773986, 31.50000000000000000, 13.85410196624972201 ) ) ;
#19308=CIRCLE ( 'NONE', #10963, 6.000000000000000000 ) ;
#19315=CARTESIAN_POINT ( 'NONE',  ( -1.878215178124994722, 25.40312499938548996, 5.746835883940462963 ) ) ;
#19320=ORIENTED_EDGE ( 'NONE', *, *, #22473, .F. ) ;
#19324=CARTESIAN_POINT ( 'NONE',  ( 3.526711513754818395, 31.50000000000000000, 4.145898033750289535 ) ) ;
#19325=CARTESIAN_POINT ( 'NONE',  ( 4.006172263299091013E-15, 26.71562499938548996, 4.662447845253954171 ) ) ;
#19327=B_SPLINE_CURVE_WITH_KNOTS ( 'NONE', 3,
 ( #7951, #5858, #2207, #13975, #8089, #11874, #17766, #24293, #3903, #14368, #19841, #25735, #18033, #1942, #9904, #21944 ),
 .UNSPECIFIED., .F., .F.,
 ( 4, 2, 2, 2, 2, 2, 2, 4 ),
 ( 2.789812634921229689E-07, 0.0002085651107750574140, 0.0004168512402866226684, 0.0006251373697981880582, 0.0008334234993097532854, 0.001041709628821318621, 0.001249995758332883957, 0.001666568017356004870 ),
 .UNSPECIFIED. ) ;
#19345=CARTESIAN_POINT ( 'NONE',  ( 3.756430356250004987, 29.75312499938549138, 8.999999999999992895 ) ) ;
#19368=CARTESIAN_POINT ( 'NONE',  ( -5.706339097770933400, 38.63519838069944967, 7.645898033750358813 ) ) ;
#19376=DIRECTION ( 'NONE',  ( -0.000000000000000000, -1.000000000000000000, -0.000000000000000000 ) ) ;
#19379=CARTESIAN_POINT ( 'NONE',  ( -3.526711513754773986, 29.50000000000000000, 13.85410196624972201 ) ) ;
#19388=CARTESIAN_POINT ( 'NONE',  ( 4.000000000000002665, 29.46250000000000568, 11.30940107675849760 ) ) ;
#19390=CARTESIAN_POINT ( 'NONE',  ( -1.071796769724489895, 25.76740381056767148, 12.99999999999999289 ) ) ;
#19402=CARTESIAN_POINT ( 'NONE',  ( 4.000000000000002665, 28.50624999877097210, 11.30940107675849760 ) ) ;
#19414=CARTESIAN_POINT ( 'NONE',  ( 3.756430356250000546, 29.15312499938548996, 11.16877607737301403 ) ) ;
#19416=CARTESIAN_POINT ( 'NONE',  ( 6.009258394948636914E-15, 26.46250000000000213, 4.381197846482986158 ) ) ;
#19417=ADVANCED_FACE ( 'NONE', ( #3386 ), #11104, .F. ) ;
#19425=DIRECTION ( 'NONE',  ( -0.000000000000000000, 1.000000000000000000, -0.000000000000000000 ) ) ;
#19428=CARTESIAN_POINT ( 'NONE',  ( -7.901901826148023498E-15, 28.71250000000000568, 4.999999999999992006 ) ) ;
#19444=CARTESIAN_POINT ( 'NONE',  ( 3.756430356250004543, 29.71562499938548996, 11.16877607737301226 ) ) ;
#19477=CARTESIAN_POINT ( 'NONE',  ( 3.756430356250002323, 25.62812499938548072, 6.831223922626973533 ) ) ;
#19481=DIRECTION ( 'NONE',  ( 0.000000000000000000, 0.000000000000000000, 1.000000000000000000 ) ) ;
#19496=VERTEX_POINT ( 'NONE', #17508 ) ;
#19498=ORIENTED_EDGE ( 'NONE', *, *, #10685, .F. ) ;
#19501=CARTESIAN_POINT ( 'NONE',  ( 3.469446951953614189E-15, 35.50000000000000711, 8.999999999999992895 ) ) ;
#19517=CARTESIAN_POINT ( 'NONE',  ( 4.000000000000003553, 27.64374999877097139, 8.999999999999992895 ) ) ;
#19528=CARTESIAN_POINT ( 'NONE',  ( 3.434593913234900153, 38.94978637201472793, 4.639884373247868510 ) ) ;
#19530=CARTESIAN_POINT ( 'NONE',  ( -1.878215178124994722, 27.99062499938548143, 5.746835883940462963 ) ) ;
#19533=CARTESIAN_POINT ( 'NONE',  ( -3.999999999999996447, 26.08750000000000213, 6.690598923241487306 ) ) ;
#19537=EDGE_CURVE ( 'NONE', #17035, #23841, #18038, .T. ) ;
#19543=DIRECTION ( 'NONE',  ( 0.000000000000000000, 1.000000000000000000, 0.000000000000000000 ) ) ;
#19548=CARTESIAN_POINT ( 'NONE',  ( 4.000000000000005329, 25.88124999877097565, 6.690598923241489970 ) ) ;
#19550=ORIENTED_EDGE ( 'NONE', *, *, #23567, .T. ) ;
#19554=CARTESIAN_POINT ( 'NONE',  ( 4.006172263299091013E-15, 25.36562499938549564, 4.662447845253954171 ) ) ;
#19563=DIRECTION ( 'NONE',  ( 0.000000000000000000, 0.000000000000000000, -1.000000000000000000 ) ) ;
#19564=CARTESIAN_POINT ( 'NONE',  ( -3.756430356250000546, 29.56562499938549493, 11.16877607737301226 ) ) ;
#19586=EDGE_CURVE ( 'NONE', #12207, #4893, #17933, .T. ) ;
#19590=CARTESIAN_POINT ( 'NONE',  ( 1.071796769724497222, 28.45134618820330275, 12.99999999999998757 ) ) ;
#19593=EDGE_CURVE ( 'NONE', #17035, #18497, #1899, .T. ) ;
#19602=FACE_OUTER_BOUND ( 'NONE', #24615, .T. ) ;
#19624=CARTESIAN_POINT ( 'NONE',  ( -9.296355089585910693E-16, 26.91250000000000497, 4.999999999999991118 ) ) ;
#19633=CYLINDRICAL_SURFACE ( 'NONE', #518, 4.000000000000000000 ) ;
#19645=CARTESIAN_POINT ( 'NONE',  ( -4.000000000000000000, 27.41874999877096997, 8.999999999999992895 ) ) ;
#19647=FACE_OUTER_BOUND ( 'NONE', #6005, .T. ) ;
#19655=CARTESIAN_POINT ( 'NONE',  ( 3.756430356250004543, 25.29062499938548925, 6.831223922626973533 ) ) ;
#19664=VECTOR ( 'NONE', #656, 1000.000000000000000 ) ;
#19670=CARTESIAN_POINT ( 'NONE',  ( 3.756430356250004099, 27.87812499938548783, 6.831223922626973533 ) ) ;
#19675=CARTESIAN_POINT ( 'NONE',  ( -3.999999999999994671, 26.98750000000000782, 6.690598923241487306 ) ) ;
#19680=VECTOR ( 'NONE', #10556, 1000.000000000000000 ) ;
#19689=CARTESIAN_POINT ( 'NONE',  ( 2.000000000000003553, 27.26874999877097494, 5.535898384862238508 ) ) ;
#19691=CYLINDRICAL_SURFACE ( 'NONE', #18817, 4.000000000000000000 ) ;
#19705=CARTESIAN_POINT ( 'NONE',  ( 1.878215178124998275, 25.51562499938548711, 12.25316411605952283 ) ) ;
#19706=AXIS2_PLACEMENT_3D ( 'NONE', #24989, #10859, #24742 ) ;
#19709=EDGE_CURVE ( 'NONE', #17641, #345, #4555, .T. ) ;
#19729=CARTESIAN_POINT ( 'NONE',  ( -3.999999999999996447, 26.16250000000000497, 11.30940107675849404 ) ) ;
#19730=PLANE ( 'NONE',  #2639 ) ;
#19732=CARTESIAN_POINT ( 'NONE',  ( 0.000000000000000000, 29.64062499938549422, 13.33755215474602984 ) ) ;
#19735=ORIENTED_EDGE ( 'NONE', *, *, #23772, .T. ) ;
#19743=( NAMED_UNIT ( * ) SI_UNIT ( $, .STERADIAN. ) SOLID_ANGLE_UNIT ( ) );
#19744=CARTESIAN_POINT ( 'NONE',  ( -3.756430356249996105, 27.12812499938548783, 6.831223922626973533 ) ) ;
#19761=CARTESIAN_POINT ( 'NONE',  ( 3.918623196469464443, 34.50000000000000000, 4.456389954662532737 ) ) ;
#19763=DIRECTION ( 'NONE',  ( -0.000000000000000000, 1.000000000000000000, -0.000000000000000000 ) ) ;
#19767=( BOUNDED_CURVE ( )  B_SPLINE_CURVE ( 2, ( #1152, #25342, #25606, #15409, #3124, #1545, #21166, #7422, #23382 ),
 .UNSPECIFIED., .F., .F. ) 
 B_SPLINE_CURVE_WITH_KNOTS ( ( 3, 2, 2, 2, 3 ),
 ( 0.3750000000000000000, 0.3833333333333333592, 0.4000000000000000222, 0.4166666666666666852, 0.4250000000000000444 ),
 .UNSPECIFIED. ) 
 CURVE ( )  GEOMETRIC_REPRESENTATION_ITEM ( )  RATIONAL_B_SPLINE_CURVE ( ( 0.9330127018922194093, 0.9330127018922194093, 1.000000000000000000, 0.8660254037844387076, 1.000000000000000000, 0.8660254037844387076, 1.000000000000000000, 0.9330127018922191873, 0.9330127018922194093 ) ) 
 REPRESENTATION_ITEM ( '' )  );
#19768=ORIENTED_EDGE ( 'NONE', *, *, #9599, .F. ) ;
#19772=VERTEX_POINT ( 'NONE', #25833 ) ;
#19777=CARTESIAN_POINT ( 'NONE',  ( 1.859271017917182139E-15, 29.38750000000000639, 12.99999999999999289 ) ) ;
#19779=CARTESIAN_POINT ( 'NONE',  ( 1.071796769724495446, 25.99240381056766935, 4.999999999999992895 ) ) ;
#19783=CARTESIAN_POINT ( 'NONE',  ( 3.959305671612554781E-15, 31.50000000000000000, 12.99999999999999289 ) ) ;
#19789=CARTESIAN_POINT ( 'NONE',  ( 1.878215178125001605, 26.07812499938549067, 12.25316411605952283 ) ) ;
#19795=EDGE_LOOP ( 'NONE', ( #1383, #17696 ) ) ;
#19796=VERTEX_POINT ( 'NONE', #5823 ) ;
#19797=CARTESIAN_POINT ( 'NONE',  ( -1.071796769724488785, 26.16115380933863577, 12.99999999999999289 ) ) ;
#19799=CARTESIAN_POINT ( 'NONE',  ( 0.4972522109372495280, 38.55547752541761497, 14.92368914124902801 ) ) ;
#19801=CARTESIAN_POINT ( 'NONE',  ( -3.756430356249994773, 27.16562499938548214, 8.999999999999992895 ) ) ;
#19803=CARTESIAN_POINT ( 'NONE',  ( 4.000000000000001776, 25.90000000000000568, 8.999999999999992895 ) ) ;
#19813=CARTESIAN_POINT ( 'NONE',  ( -4.648177544792955347E-16, 27.08124999877097139, 12.99999999999999289 ) ) ;
#19815=DIRECTION ( 'NONE',  ( 0.000000000000000000, 0.000000000000000000, -1.000000000000000000 ) ) ;
#19819=CARTESIAN_POINT ( 'NONE',  ( 3.756430356250004099, 25.29062499938548925, 6.831223922626973533 ) ) ;
#19827=CARTESIAN_POINT ( 'NONE',  ( -1.878215178124994722, 25.29062499938548925, 5.746835883940462963 ) ) ;
#19841=CARTESIAN_POINT ( 'NONE',  ( 5.242549070241824261, 39.00275152493676245, 7.344768029949470645 ) ) ;
#19844=EDGE_CURVE ( 'NONE', #11111, #10619, #10375, .T. ) ;
#19846=CARTESIAN_POINT ( 'NONE',  ( 3.017230054654504556, 38.72260848564139479, 13.92749297489922355 ) ) ;
#19860=CARTESIAN_POINT ( 'NONE',  ( -3.756430356250000546, 26.30312499938548854, 11.16877607737301226 ) ) ;
#19869=CARTESIAN_POINT ( 'NONE',  ( 1.071796769724490783, 26.20134618820330630, 12.99999999999999467 ) ) ;
#19879=ORIENTED_EDGE ( 'NONE', *, *, #5087, .F. ) ;
#19882=VERTEX_POINT ( 'NONE', #24512 ) ;
#19884=EDGE_CURVE ( 'NONE', #3918, #25139, #13417, .T. ) ;
#19894=CARTESIAN_POINT ( 'NONE',  ( -1.394453263437886604E-15, 27.30624999877096926, 4.999999999999991118 ) ) ;
#19903=CARTESIAN_POINT ( 'NONE',  ( -1.878215178124998275, 26.30312499938548854, 5.746835883940462963 ) ) ;
#19915=CARTESIAN_POINT ( 'NONE',  ( 3.020711573345385315, 38.79236218548354032, 4.157123895590975060 ) ) ;
#19920=CARTESIAN_POINT ( 'NONE',  ( 6.009258394948636914E-15, 28.26250000000000639, 4.381197846482986158 ) ) ;
#19937=CARTESIAN_POINT ( 'NONE',  ( -1.878215178124998275, 27.35312499938548925, 12.25316411605951927 ) ) ;
#19947=CARTESIAN_POINT ( 'NONE',  ( -3.756430356249996549, 26.71562499938548996, 8.999999999999992895 ) ) ;
#19954=CARTESIAN_POINT ( 'NONE',  ( 3.469446951953614189E-15, 38.49999999999999289, 8.999999999999992895 ) ) ;
#19955=CARTESIAN_POINT ( 'NONE',  ( 4.000000000000005329, 29.48124999877097707, 6.690598923241489970 ) ) ;
#19962=CARTESIAN_POINT ( 'NONE',  ( -5.345872705005824344, 38.71721868403346178, 11.20510013807279037 ) ) ;
#19966=CARTESIAN_POINT ( 'NONE',  ( -1.999999999999994893, 26.05000000000000426, 5.535898384862237620 ) ) ;
#19967=FACE_OUTER_BOUND ( 'NONE', #12528, .T. ) ;
#19980=CIRCLE ( 'NONE', #3708, 0.5000000000000004441 ) ;
#19984=CARTESIAN_POINT ( 'NONE',  ( -3.756430356249994773, 27.16562499938548214, 8.999999999999992895 ) ) ;
#19991=CYLINDRICAL_SURFACE ( 'NONE', #15540, 4.000000000000000000 ) ;
#19997=CARTESIAN_POINT ( 'NONE',  ( 2.000000000000000000, 27.62500000000000355, 12.46410161513774817 ) ) ;
#20015=DIRECTION ( 'NONE',  ( 0.000000000000000000, 0.000000000000000000, -1.000000000000000000 ) ) ;
#20035=FACE_OUTER_BOUND ( 'NONE', #17781, .T. ) ;
#20040=CARTESIAN_POINT ( 'NONE',  ( 1.878215178125003382, 26.67812499938548854, 5.746835883940462963 ) ) ;
#20045=CARTESIAN_POINT ( 'NONE',  ( -1.071796769724487230, 28.28259618943233988, 4.999999999999992006 ) ) ;
#20056=CARTESIAN_POINT ( 'NONE',  ( -3.999999999999996447, 29.23750000000000782, 6.690598923241487306 ) ) ;
#20061=AXIS2_PLACEMENT_3D ( 'NONE', #6452, #14554, #12208 ) ;
#20075=CARTESIAN_POINT ( 'NONE',  ( -3.756430356249994329, 26.79062499938548925, 6.831223922626973533 ) ) ;
#20085=CARTESIAN_POINT ( 'NONE',  ( -2.003086131649545506E-15, 26.82812499938549067, 13.33755215474602984 ) ) ;
#20088=AXIS2_PLACEMENT_3D ( 'NONE', #8604, #14880, #10679 ) ;
#20096=CARTESIAN_POINT ( 'NONE',  ( 4.000000000000005329, 29.44374999877097210, 8.999999999999992895 ) ) ;
#20106=AXIS2_PLACEMENT_3D ( 'NONE', #13953, #6454, #13683 ) ;
#20107=CARTESIAN_POINT ( 'NONE',  ( -1.999999999999994893, 29.14374999877097139, 5.535898384862237620 ) ) ;
#20122=CARTESIAN_POINT ( 'NONE',  ( -3.756430356249996105, 26.34062499938548285, 6.831223922626973533 ) ) ;
#20124=CARTESIAN_POINT ( 'NONE',  ( -2.003086131649545506E-15, 26.82812499938549067, 13.33755215474602984 ) ) ;
#20140=CARTESIAN_POINT ( 'NONE',  ( -1.998723687422152831E-12, 39.00000000001113420, 14.49999999998978240 ) ) ;
#20154=ORIENTED_EDGE ( 'NONE', *, *, #3296, .F. ) ;
#20172=CARTESIAN_POINT ( 'NONE',  ( 0.000000000000000000, 27.84062499938548996, 13.33755215474602984 ) ) ;
#20174=EDGE_LOOP ( 'NONE', ( #333, #5559 ) ) ;
#20179=CONICAL_SURFACE ( 'NONE', #11004, 5.000000000000000888, 0.7853981633974445042 ) ;
#20180=CARTESIAN_POINT ( 'NONE',  ( -3.999999999999999112, 26.10624999877097707, 11.30940107675849404 ) ) ;
#20182=EDGE_CURVE ( 'NONE', #16757, #11943, #9996, .T. ) ;
#20186=DIRECTION ( 'NONE',  ( 0.000000000000000000, 1.000000000000000000, 0.000000000000000000 ) ) ;
#20188=CARTESIAN_POINT ( 'NONE',  ( 0.000000000000000000, 28.48750000000000426, 13.61880215351699874 ) ) ;
#20202=CARTESIAN_POINT ( 'NONE',  ( 2.003086131649545506E-15, 26.94062499938549138, 13.33755215474603162 ) ) ;
#20207=DIRECTION ( 'NONE',  ( 0.000000000000000000, 1.000000000000000000, -0.000000000000000000 ) ) ;
#20213=CARTESIAN_POINT ( 'NONE',  ( 8.012344526598182026E-15, 27.05312499938548854, 4.662447845253954171 ) ) ;
#20219=DIRECTION ( 'NONE',  ( 0.000000000000000000, 0.000000000000000000, -1.000000000000000000 ) ) ;
#20236=ORIENTED_EDGE ( 'NONE', *, *, #11708, .T. ) ;
#20239=CARTESIAN_POINT ( 'NONE',  ( 3.253724281355068545E-15, 25.50624999877097210, 4.999999999999992006 ) ) ;
#20240=ORIENTED_EDGE ( 'NONE', *, *, #25688, .T. ) ;
#20244=ORIENTED_EDGE ( 'NONE', *, *, #1611, .T. ) ;
#20247=CARTESIAN_POINT ( 'NONE',  ( -3.756430356249994773, 26.37812499938548783, 8.999999999999992895 ) ) ;
#20262=CARTESIAN_POINT ( 'NONE',  ( 9.296355089585910693E-16, 26.18124999877097281, 12.99999999999999289 ) ) ;
#20267=CARTESIAN_POINT ( 'NONE',  ( 2.000000000000000000, 27.56874999877097210, 12.46410161513774817 ) ) ;
#20276=EDGE_CURVE ( 'NONE', #25560, #23884, #24233, .T. ) ;
#20292=( BOUNDED_CURVE ( )  B_SPLINE_CURVE ( 2, ( #3612, #19819, #11581, #19554, #19315, #3493, #9763, #7672, #23623, #9633, #11719, #13442, #5701, #1410, #13680, #17364, #17867, #17611, #5829, #25588, #21653, #7409, #25839, #17742, #13816, #7922, #15909, #5967, #21412, #2178, #10139, #16557, #18143, #12100, #12362, #8064, #4121, #20457, #3999, #18003, #14203, #20075, #10009, #22305, #216, #20202, #6088, #11966, #18522, #4382, #10525, #92, #8186, #12235, #2041, #16046, #19937, #16164, #24127, #609, #6350, #8576, #16296, #24008, #24516, #6213, #2556, #4261, #13950, #14072, #21918, #8448, #22176, #2303, #8310, #10259, #479, #18253, #14463, #22038, #336, #24263, #14343, #20327, #2417, #10379, #18379, #16437, #24401, #6477, #22426, #4506, #12484, #16944, #1106, #2944, #6869, #14973, #20999, #18642, #6989, #7127, #12758, #3076, #22704, #2808, #6599, #6735, #8969, #4901, #10910, #22951, #4784, #25039, #20730, #20601, #24913, #10772, #11042, #14585, #4648 ),
 .UNSPECIFIED., .F., .F. ) 
 B_SPLINE_CURVE_WITH_KNOTS ( ( 3, 2, 2, 2, 2, 2, 2, 2, 2, 2, 2, 2, 2, 2, 2, 2, 2, 2, 2, 2, 2, 2, 2, 2, 2, 2, 2, 2, 2, 2, 2, 2, 2, 2, 2, 2, 2, 2, 2, 2, 2, 2, 2, 2, 2, 2, 2, 2, 2, 2, 2, 2, 2, 2, 2, 2, 2, 2, 2, 2, 3 ),
 ( 0.000000000000000000, 0.01666666666666666644, 0.03333333333333333287, 0.05000000000000000278, 0.06666666666666666574, 0.08333333333333332871, 0.1000000000000000056, 0.1166666666666666685, 0.1333333333333333315, 0.1499999999999999944, 0.1666666666666666574, 0.1833333333333333204, 0.2000000000000000111, 0.2166666666666666741, 0.2333333333333333370, 0.2500000000000000000, 0.2666666666666666630, 0.2833333333333333259, 0.2999999999999999889, 0.3166666666666666519, 0.3333333333333333148, 0.3499999999999999778, 0.3666666666666666408, 0.3833333333333333592, 0.4000000000000000222, 0.4166666666666666852, 0.4333333333333333481, 0.4500000000000000111, 0.4666666666666666741, 0.4833333333333333370, 0.5000000000000000000, 0.5166666666666667185, 0.5333333333333333259, 0.5500000000000000444, 0.5666666666666666519, 0.5833333333333333703, 0.5999999999999999778, 0.6166666666666666963, 0.6333333333333333037, 0.6500000000000000222, 0.6666666666666666297, 0.6833333333333333481, 0.6999999999999999556, 0.7166666666666666741, 0.7333333333333332815, 0.7500000000000000000, 0.7666666666666667185, 0.7833333333333333259, 0.8000000000000000444, 0.8166666666666666519, 0.8333333333333333703, 0.8499999999999999778, 0.8666666666666666963, 0.8833333333333333037, 0.9000000000000000222, 0.9166666666666666297, 0.9333333333333333481, 0.9499999999999999556, 0.9666666666666666741, 0.9833333333333332815, 1.000000000000000000 ),
 .UNSPECIFIED. ) 
 CURVE ( )  GEOMETRIC_REPRESENTATION_ITEM ( )  RATIONAL_B_SPLINE_CURVE ( ( 1.000000000000000000, 0.8660254037844387076, 1.000000000000000000, 0.8660254037844387076, 1.000000000000000000, 0.8660254037844387076, 1.000000000000000000, 0.8660254037844387076, 1.000000000000000000, 0.8660254037844387076, 1.000000000000000000, 0.8660254037844387076, 1.000000000000000000, 0.8660254037844387076, 1.000000000000000000, 0.8660254037844387076, 1.000000000000000000, 0.8660254037844387076, 1.000000000000000000, 0.8660254037844387076, 1.000000000000000000, 0.8660254037844387076, 1.000000000000000000, 0.8660254037844387076, 1.000000000000000000, 0.8660254037844387076, 1.000000000000000000, 0.8660254037844387076, 1.000000000000000000, 0.8660254037844387076, 1.000000000000000000, 0.8660254037844387076, 1.000000000000000000, 0.8660254037844387076, 1.000000000000000000, 0.8660254037844387076, 1.000000000000000000, 0.8660254037844387076, 1.000000000000000000, 0.8660254037844387076, 1.000000000000000000, 0.8660254037844387076, 1.000000000000000000, 0.8660254037844387076, 1.000000000000000000, 0.8660254037844387076, 1.000000000000000000, 0.8660254037844387076, 1.000000000000000000, 0.8660254037844387076, 1.000000000000000000, 0.8660254037844387076, 1.000000000000000000, 0.8660254037844387076, 1.000000000000000000, 0.8660254037844387076, 1.000000000000000000, 0.8660254037844387076, 1.000000000000000000, 0.8660254037844387076, 1.000000000000000000, 0.8660254037844387076, 1.000000000000000000, 0.8660254037844387076, 1.000000000000000000, 0.8660254037844387076, 1.000000000000000000, 0.8660254037844387076, 1.000000000000000000, 0.8660254037844387076, 1.000000000000000000, 0.8660254037844387076, 1.000000000000000000, 0.8660254037844387076, 1.000000000000000000, 0.8660254037844387076, 1.000000000000000000, 0.8660254037844387076, 1.000000000000000000, 0.8660254037844387076, 1.000000000000000000, 0.8660254037844387076, 1.000000000000000000, 0.8660254037844387076, 1.000000000000000000, 0.8660254037844387076, 1.000000000000000000, 0.8660254037844387076, 1.000000000000000000, 0.8660254037844387076, 1.000000000000000000, 0.8660254037844387076, 1.000000000000000000, 0.8660254037844387076, 1.000000000000000000, 0.8660254037844387076, 1.000000000000000000, 0.8660254037844387076, 1.000000000000000000, 0.8660254037844387076, 1.000000000000000000, 0.8660254037844387076, 1.000000000000000000, 0.8660254037844387076, 1.000000000000000000, 0.8660254037844387076, 1.000000000000000000, 0.8660254037844387076, 1.000000000000000000, 0.8660254037844387076, 1.000000000000000000, 0.8660254037844387076, 1.000000000000000000, 0.8660254037844387076, 1.000000000000000000, 0.8660254037844387076, 1.000000000000000000, 0.8660254037844387076, 1.000000000000000000, 0.8660254037844387076, 1.000000000000000000 ) ) 
 REPRESENTATION_ITEM ( '' )  );
#20296=ORIENTED_EDGE ( 'NONE', *, *, #6858, .T. ) ;
#20298=CARTESIAN_POINT ( 'NONE',  ( 1.878215178125005158, 27.12812499938548783, 5.746835883940462963 ) ) ;
#20306=DIRECTION ( 'NONE',  ( -0.000000000000000000, 1.000000000000000000, -0.000000000000000000 ) ) ;
#20309=ADVANCED_FACE ( 'NONE', ( #6450 ), #10493, .T. ) ;
#20312=CARTESIAN_POINT ( 'NONE',  ( -3.999999999999999556, 29.31250000000000000, 11.30940107675849404 ) ) ;
#20323=DIRECTION ( 'NONE',  ( 0.000000000000000000, -1.000000000000000000, 0.000000000000000000 ) ) ;
#20327=CARTESIAN_POINT ( 'NONE',  ( 3.756430356250000546, 28.36562499938548854, 11.16877607737301403 ) ) ;
#20331=CARTESIAN_POINT ( 'NONE',  ( 6.938893903907228378E-15, 29.50000000000000000, 3.499999999999992450 ) ) ;
#20336=CARTESIAN_POINT ( 'NONE',  ( 1.878215178124998275, 28.21562499938549351, 12.25316411605952283 ) ) ;
#20354=ORIENTED_EDGE ( 'NONE', *, *, #12171, .F. ) ;
#20368=CARTESIAN_POINT ( 'NONE',  ( -3.753948939949354635, 38.72260848564138769, 13.39223537354781080 ) ) ;
#20391=ORIENTED_EDGE ( 'NONE', *, *, #19884, .T. ) ;
#20392=ORIENTED_EDGE ( 'NONE', *, *, #21512, .T. ) ;
#20400=CYLINDRICAL_SURFACE ( 'NONE', #17780, 6.000000000000000888 ) ;
#20408=CYLINDRICAL_SURFACE ( 'NONE', #24231, 4.000000000000000000 ) ;
#20418=EDGE_LOOP ( 'NONE', ( #25325, #6668, #6323 ) ) ;
#20420=CARTESIAN_POINT ( 'NONE',  ( -1.878215178124996498, 28.55312499938548854, 5.746835883940462963 ) ) ;
#20441=CARTESIAN_POINT ( 'NONE',  ( 4.000000000000002665, 29.46250000000000568, 11.30940107675849760 ) ) ;
#20457=CARTESIAN_POINT ( 'NONE',  ( 3.756430356250004099, 26.64062499938549422, 6.831223922626973533 ) ) ;
#20459=ORIENTED_EDGE ( 'NONE', *, *, #7590, .T. ) ;
#20469=CARTESIAN_POINT ( 'NONE',  ( -3.756430356249996105, 27.57812499938548356, 6.831223922626973533 ) ) ;
#20504=VERTEX_POINT ( 'NONE', #11136 ) ;
#20506=ORIENTED_EDGE ( 'NONE', *, *, #11274, .F. ) ;
#20511=CARTESIAN_POINT ( 'NONE',  ( -3.756430356249998326, 25.51562499938549067, 11.16877607737301226 ) ) ;
#20525=DIRECTION ( 'NONE',  ( 0.000000000000000000, 1.000000000000000000, 0.000000000000000000 ) ) ;
#20538=CIRCLE ( 'NONE', #21384, 6.000000000000000000 ) ;
#20563=CARTESIAN_POINT ( 'NONE',  ( 6.972266317189432034E-15, 28.65624999877097423, 4.999999999999992006 ) ) ;
#20570=CARTESIAN_POINT ( 'NONE',  ( 1.878215178124999829, 28.32812499938549422, 12.25316411605952283 ) ) ;
#20571=VECTOR ( 'NONE', #16643, 1000.000000000000000 ) ;
#20575=CARTESIAN_POINT ( 'NONE',  ( -3.999999999999996447, 28.33750000000000568, 6.690598923241487306 ) ) ;
#20577=CARTESIAN_POINT ( 'NONE',  ( -3.999999999999996447, 27.83124999877097139, 6.690598923241487306 ) ) ;
#20580=CARTESIAN_POINT ( 'NONE',  ( -0.4995657836784084815, 34.50000000000000000, 14.97916666666665897 ) ) ;
#20583=ADVANCED_FACE ( 'NONE', ( #17037 ), #13120, .T. ) ;
#20594=CARTESIAN_POINT ( 'NONE',  ( 0.000000000000000000, 26.18124999877096926, 13.61880215351699874 ) ) ;
#20601=CARTESIAN_POINT ( 'NONE',  ( -3.756430356250000546, 29.56562499938549493, 11.16877607737301048 ) ) ;
#20606=CARTESIAN_POINT ( 'NONE',  ( 3.959305671612554781E-15, 35.50000000000000711, 12.99999999999999289 ) ) ;
#20614=CARTESIAN_POINT ( 'NONE',  ( 0.000000000000000000, 27.72812499938548925, 13.33755215474602984 ) ) ;
#20633=VERTEX_POINT ( 'NONE', #15989 ) ;
#20646=CARTESIAN_POINT ( 'NONE',  ( -3.849711841530632839, 38.61087488181074434, 13.45662818444764497 ) ) ;
#20648=ADVANCED_FACE ( 'NONE', ( #13374 ), #3674, .F. ) ;
#20660=CYLINDRICAL_SURFACE ( 'NONE', #21394, 0.5000000000000004441 ) ;
#20667=ORIENTED_EDGE ( 'NONE', *, *, #7657, .T. ) ;
#20669=DIRECTION ( 'NONE',  ( 0.000000000000000000, -1.000000000000000000, 0.000000000000000000 ) ) ;
#20698=CARTESIAN_POINT ( 'NONE',  ( 3.756430356250004543, 27.54062499938548925, 6.831223922626973533 ) ) ;
#20704=CARTESIAN_POINT ( 'NONE',  ( -5.840899737312954976, 34.50000000000000000, 10.37254881831481512 ) ) ;
#20705=EDGE_LOOP ( 'NONE', ( #1983, #2109, #15357, #93 ) ) ;
#20723=CARTESIAN_POINT ( 'NONE',  ( 2.000000000000003553, 26.36874999877097281, 5.535898384862238508 ) ) ;
#20730=CARTESIAN_POINT ( 'NONE',  ( -3.756430356249996549, 29.52812499938548996, 8.999999999999992895 ) ) ;
#20739=CARTESIAN_POINT ( 'NONE',  ( 6.009258394948636914E-15, 26.60312499938547859, 4.662447845253954171 ) ) ;
#20741=CARTESIAN_POINT ( 'NONE',  ( 1.071796769724494114, 26.25759618943234130, 12.99999999999999112 ) ) ;
#20742=CARTESIAN_POINT ( 'NONE',  ( 4.006172263299091013E-15, 25.11250000000000426, 4.381197846482986158 ) ) ;
#20743=DIRECTION ( 'NONE',  ( 0.000000000000000000, 0.000000000000000000, 1.000000000000000000 ) ) ;
#20765=CARTESIAN_POINT ( 'NONE',  ( 1.071796769724489895, 29.80134618820331127, 12.99999999999999467 ) ) ;
#20771=ORIENTED_EDGE ( 'NONE', *, *, #9258, .F. ) ;
#20773=CARTESIAN_POINT ( 'NONE',  ( 3.756430356250006319, 27.99062499938548854, 6.831223922626973533 ) ) ;
#20780=CARTESIAN_POINT ( 'NONE',  ( 3.918623196469491088, 34.50000000000000000, 13.54361004533742907 ) ) ;
#20794=EDGE_CURVE ( 'NONE', #25495, #12364, #19980, .T. ) ;
#20802=CIRCLE ( 'NONE', #21224, 4.000000000000000000 ) ;
#20830=AXIS2_PLACEMENT_3D ( 'NONE', #23140, #5340, #5219 ) ;
#20840=EDGE_CURVE ( 'NONE', #12137, #14315, #12584, .T. ) ;
#20858=CARTESIAN_POINT ( 'NONE',  ( 2.000000000000003553, 27.32500000000000995, 5.535898384862238508 ) ) ;
#20867=CARTESIAN_POINT ( 'NONE',  ( 1.878215178124998275, 28.21562499938549351, 12.25316411605952283 ) ) ;
#20902=CARTESIAN_POINT ( 'NONE',  ( -3.756430356249994329, 28.59062499938548996, 6.831223922626973533 ) ) ;
#20943=LINE ( 'NONE', #10855, #7750 ) ;
#20951=FACE_OUTER_BOUND ( 'NONE', #3777, .T. ) ;
#20975=VERTEX_POINT ( 'NONE', #15010 ) ;
#20983=B_SPLINE_CURVE_WITH_KNOTS ( 'NONE', 3,
 ( #2422, #4386, #12367, #6481, #8454, #10142 ),
 .UNSPECIFIED., .F., .F.,
 ( 4, 2, 4 ),
 ( 0.001259672601285470291, 0.001557997829463299462, 0.001856323057641128850 ),
 .UNSPECIFIED. ) ;
#20987=VECTOR ( 'NONE', #25854, 1000.000000000000000 ) ;
#20993=CARTESIAN_POINT ( 'NONE',  ( 4.000000000000005329, 28.05624999877097281, 11.30940107675849760 ) ) ;
#20998=ADVANCED_FACE ( 'NONE', ( #12365 ), #2691, .T. ) ;
#20999=CARTESIAN_POINT ( 'NONE',  ( 1.878215178125008489, 28.92812499938549209, 5.746835883940462963 ) ) ;
#21004=CARTESIAN_POINT ( 'NONE',  ( 5.112995299272250684E-15, 27.36250000000000426, 4.999999999999992006 ) ) ;
#21008=CARTESIAN_POINT ( 'NONE',  ( 4.006172263299091013E-15, 25.70312499938548356, 4.662447845253954171 ) ) ;
#21011=CARTESIAN_POINT ( 'NONE',  ( 4.006172263299091013E-15, 25.56250000000000711, 4.381197846482986158 ) ) ;
#21013=CARTESIAN_POINT ( 'NONE',  ( 3.469446951953614189E-15, 38.49999999999999289, 8.999999999999992895 ) ) ;
#21015=CYLINDRICAL_SURFACE ( 'NONE', #2069, 4.000000000000000000 ) ;
#21022=DIRECTION ( 'NONE',  ( 0.000000000000000000, 0.000000000000000000, 1.000000000000000000 ) ) ;
#21027=VERTEX_POINT ( 'NONE', #16824 ) ;
#21032=LINE ( 'NONE', #5203, #9184 ) ;
#21036=AXIS2_PLACEMENT_3D ( 'NONE', #13353, #15703, #13223 ) ;
#21043=CARTESIAN_POINT ( 'NONE',  ( -1.878215178124994722, 26.75312499938549138, 5.746835883940462963 ) ) ;
#21049=CARTESIAN_POINT ( 'NONE',  ( 1.071796769724490783, 28.95759618943234059, 12.99999999999999467 ) ) ;
#21052=CARTESIAN_POINT ( 'NONE',  ( 3.878215178125005380, 29.57031249969274356, 8.999999999999992895 ) ) ;
#21063=CARTESIAN_POINT ( 'NONE',  ( -4.648177544792955347E-16, 26.85624999877096997, 4.999999999999991118 ) ) ;
#21066=ORIENTED_EDGE ( 'NONE', *, *, #15240, .F. ) ;
#21067=ORIENTED_EDGE ( 'NONE', *, *, #24600, .F. ) ;
#21097=ORIENTED_EDGE ( 'NONE', *, *, #18233, .T. ) ;
#21110=CARTESIAN_POINT ( 'NONE',  ( -1.999999999999998224, 28.84374999877097423, 12.46410161513774639 ) ) ;
#21122=CARTESIAN_POINT ( 'NONE',  ( 0.000000000000000000, 29.52812499938548640, 13.33755215474602984 ) ) ;
#21123=CARTESIAN_POINT ( 'NONE',  ( 5.532151103383248447, 38.49999999999999289, 11.32277940608563149 ) ) ;
#21127=CARTESIAN_POINT ( 'NONE',  ( -1.878215178124994722, 29.34062499938548640, 5.746835883940462963 ) ) ;
#21130=DIRECTION ( 'NONE',  ( 0.000000000000000000, 0.000000000000000000, 1.000000000000000000 ) ) ;
#21141=( BOUNDED_CURVE ( )  B_SPLINE_CURVE ( 2, ( #18869, #4867, #3283, #15206, #23174, #21204, #11255, #19239, #1341 ),
 .UNSPECIFIED., .F., .F. ) 
 B_SPLINE_CURVE_WITH_KNOTS ( ( 3, 2, 2, 2, 3 ),
 ( 0.02500000000000000139, 0.03333333333333333287, 0.05000000000000000278, 0.06666666666666666574, 0.07500000000000001110 ),
 .UNSPECIFIED. ) 
 CURVE ( )  GEOMETRIC_REPRESENTATION_ITEM ( )  RATIONAL_B_SPLINE_CURVE ( ( 0.9330127018922194093, 0.9330127018922194093, 1.000000000000000000, 0.8660254037844387076, 1.000000000000000000, 0.8660254037844387076, 1.000000000000000000, 0.9330127018922191873, 0.9330127018922192983 ) ) 
 REPRESENTATION_ITEM ( '' )  );
#21151=DIRECTION ( 'NONE',  ( 0.000000000000000000, 1.000000000000000000, -0.000000000000000000 ) ) ;
#21158=LINE ( 'NONE', #9506, #18505 ) ;
#21159=CARTESIAN_POINT ( 'NONE',  ( 0.000000000000000000, 28.29062499938548925, 13.33755215474602984 ) ) ;
#21164=DIRECTION ( 'NONE',  ( 0.000000000000000000, 0.000000000000000000, 1.000000000000000000 ) ) ;
#21166=CARTESIAN_POINT ( 'NONE',  ( 2.000000000000007105, 26.87500000000001066, 5.535898384862238508 ) ) ;
#21172=CARTESIAN_POINT ( 'NONE',  ( 3.469446951953614189E-15, 35.50000000000000711, 4.999999999999992006 ) ) ;
#21179=CARTESIAN_POINT ( 'NONE',  ( 2.003086131649545506E-15, 29.19062499938549138, 13.33755215474602984 ) ) ;
#21204=CARTESIAN_POINT ( 'NONE',  ( -3.999999999999999112, 25.26250000000000284, 11.30940107675849404 ) ) ;
#21207=ORIENTED_EDGE ( 'NONE', *, *, #9000, .T. ) ;
#21208=CARTESIAN_POINT ( 'NONE',  ( 5.112995299272250684E-15, 27.36250000000000426, 4.999999999999992006 ) ) ;
#21224=AXIS2_PLACEMENT_3D ( 'NONE', #16359, #10833, #24452 ) ;
#21231=CARTESIAN_POINT ( 'NONE',  ( 4.000000000000002665, 27.60624999877096641, 11.30940107675849760 ) ) ;
#21249=CARTESIAN_POINT ( 'NONE',  ( -3.756430356249997882, 25.85312499938549635, 11.16877607737301048 ) ) ;
#21251=CARTESIAN_POINT ( 'NONE',  ( 1.878215178125003382, 29.56562499938549138, 12.25316411605952283 ) ) ;
#21254=CARTESIAN_POINT ( 'NONE',  ( 2.000000000000003553, 29.06874999877097210, 5.535898384862238508 ) ) ;
#21255=VECTOR ( 'NONE', #114, 1000.000000000000000 ) ;
#21283=CARTESIAN_POINT ( 'NONE',  ( -3.756430356249994329, 26.86562499938548498, 11.16877607737301226 ) ) ;
#21290=SURFACE_STYLE_USAGE ( .BOTH. , #13192 ) ;
#21298=FACE_OUTER_BOUND ( 'NONE', #2662, .T. ) ;
#21312=CARTESIAN_POINT ( 'NONE',  ( 4.648177544792954952E-15, 28.26250000000000284, 4.999999999999992006 ) ) ;
#21315=VERTEX_POINT ( 'NONE', #11164 ) ;
#21325=CARTESIAN_POINT ( 'NONE',  ( -1.878215178124994722, 25.29062499938548925, 5.746835883940462963 ) ) ;
#21334=DIRECTION ( 'NONE',  ( -0.8660254037844395958, 0.4999999999999982236, 0.000000000000000000 ) ) ;
#21342=ORIENTED_EDGE ( 'NONE', *, *, #7648, .F. ) ;
#21362=ADVANCED_FACE ( 'NONE', ( #13934 ), #4369, .T. ) ;
#21375=CARTESIAN_POINT ( 'NONE',  ( 2.000000000000003553, 27.26874999877097494, 5.535898384862238508 ) ) ;
#21384=AXIS2_PLACEMENT_3D ( 'NONE', #12747, #8438, #8682 ) ;
#21388=CARTESIAN_POINT ( 'NONE',  ( 4.648177544792955347E-16, 29.33124999877097139, 12.99999999999999289 ) ) ;
#21390=CARTESIAN_POINT ( 'NONE',  ( -3.756430356249996549, 29.00312499938548427, 11.16877607737301048 ) ) ;
#21392=CYLINDRICAL_SURFACE ( 'NONE', #25640, 6.000000000000000888 ) ;
#21393=CARTESIAN_POINT ( 'NONE',  ( -1.999999999999996669, 26.20000000000000639, 12.46410161513774639 ) ) ;
#21394=AXIS2_PLACEMENT_3D ( 'NONE', #12159, #24329, #22235 ) ;
#21407=CARTESIAN_POINT ( 'NONE',  ( 3.469446951953614189E-15, 35.50000000000000711, 8.999999999999992895 ) ) ;
#21412=CARTESIAN_POINT ( 'NONE',  ( -1.878215178124998275, 26.30312499938548854, 5.746835883940462963 ) ) ;
#21421=CARTESIAN_POINT ( 'NONE',  ( -3.756430356249996549, 25.36562499938548854, 8.999999999999992895 ) ) ;
#21424=VECTOR ( 'NONE', #4622, 1000.000000000000000 ) ;
#21426=DIRECTION ( 'NONE',  ( 0.000000000000000000, -1.000000000000000000, 0.000000000000000000 ) ) ;
#21428=CARTESIAN_POINT ( 'NONE',  ( 4.000000000000002665, 29.01250000000000284, 11.30940107675849760 ) ) ;
#21435=LINE ( 'NONE', #21172, #13022 ) ;
#21444=CARTESIAN_POINT ( 'NONE',  ( 0.4995657836784084815, 38.49999999999999289, 14.97916666666666075 ) ) ;
#21450=ORIENTED_EDGE ( 'NONE', *, *, #15801, .F. ) ;
#21454=CARTESIAN_POINT ( 'NONE',  ( -3.051911138222374031, 38.91143067427094593, 13.68207702368797918 ) ) ;
#21457=( BOUNDED_CURVE ( )  B_SPLINE_CURVE ( 2, ( #8231, #16210, #4796, #24178, #6266, #22225, #4310, #8360, #12773 ),
 .UNSPECIFIED., .F., .F. ) 
 B_SPLINE_CURVE_WITH_KNOTS ( ( 3, 2, 2, 2, 3 ),
 ( 0.8250000000000000666, 0.8333333333333333703, 0.8499999999999999778, 0.8666666666666666963, 0.8750000000000000000 ),
 .UNSPECIFIED. ) 
 CURVE ( )  GEOMETRIC_REPRESENTATION_ITEM ( )  RATIONAL_B_SPLINE_CURVE ( ( 0.9330127018922194093, 0.9330127018922198534, 1.000000000000000000, 0.8660254037844387076, 1.000000000000000000, 0.8660254037844387076, 1.000000000000000000, 0.9330127018922194093, 0.9330127018922194093 ) ) 
 REPRESENTATION_ITEM ( '' )  );
#21470=CARTESIAN_POINT ( 'NONE',  ( 4.000000000000005329, 27.73750000000000782, 6.690598923241489970 ) ) ;
#21474=CYLINDRICAL_SURFACE ( 'NONE', #10795, 4.000000000000000000 ) ;
#21481=( GEOMETRIC_REPRESENTATION_CONTEXT ( 3 ) GLOBAL_UNCERTAINTY_ASSIGNED_CONTEXT ( ( #12807 ) ) GLOBAL_UNIT_ASSIGNED_CONTEXT ( ( #8621, #16989, #23003 ) ) REPRESENTATION_CONTEXT ( 'NONE', 'WORKASPACE' ) );
#21493=CARTESIAN_POINT ( 'NONE',  ( -1.071796769724487675, 27.32634618820330630, 4.999999999999992895 ) ) ;
#21500=CARTESIAN_POINT ( 'NONE',  ( 1.999999999999998224, 26.66874999877097352, 12.46410161513774817 ) ) ;
#21501=EDGE_LOOP ( 'NONE', ( #10873, #1828, #25218, #16257 ) ) ;
#21507=CARTESIAN_POINT ( 'NONE',  ( 4.000000000000001776, 25.00000000000000000, 8.999999999999992895 ) ) ;
#21510=CARTESIAN_POINT ( 'NONE',  ( 3.756430356250002323, 28.25312499938548783, 11.16877607737301403 ) ) ;
#21511=CARTESIAN_POINT ( 'NONE',  ( 6.009258394948636914E-15, 27.36250000000000782, 4.381197846482986158 ) ) ;
#21512=EDGE_CURVE ( 'NONE', #9321, #19215, #24107, .T. ) ;
#21518=AXIS2_PLACEMENT_3D ( 'NONE', #2454, #18416, #6252 ) ;
#21540=CARTESIAN_POINT ( 'NONE',  ( 1.878215178125001605, 29.22812499938549280, 12.25316411605952283 ) ) ;
#21554=CARTESIAN_POINT ( 'NONE',  ( 5.706339097771728319, 38.63519838069890966, 7.645898033751371337 ) ) ;
#21559=CARTESIAN_POINT ( 'NONE',  ( 3.048878893044081551, 38.61087488181073724, 14.03846737935104549 ) ) ;
#21565=EDGE_CURVE ( 'NONE', #22574, #12137, #711, .T. ) ;
#21569=ORIENTED_EDGE ( 'NONE', *, *, #18499, .F. ) ;
#21573=CARTESIAN_POINT ( 'NONE',  ( 1.878215178125003382, 25.66562499938548214, 5.746835883940462963 ) ) ;
#21608=CARTESIAN_POINT ( 'NONE',  ( -1.999999999999998224, 25.75000000000000711, 12.46410161513774639 ) ) ;
#21616=CARTESIAN_POINT ( 'NONE',  ( -3.999999999999996447, 29.18124999877097281, 6.690598923241487306 ) ) ;
#21620=CARTESIAN_POINT ( 'NONE',  ( -3.999999999999998224, 29.27500000000000568, 8.999999999999992895 ) ) ;
#21624=ORIENTED_EDGE ( 'NONE', *, *, #8933, .T. ) ;
#21631=CARTESIAN_POINT ( 'NONE',  ( 1.878215178125001605, 28.66562499938549280, 12.25316411605952283 ) ) ;
#21635=CARTESIAN_POINT ( 'NONE',  ( -3.999999999999996447, 27.96250000000000568, 11.30940107675849404 ) ) ;
#21640=DIRECTION ( 'NONE',  ( -0.000000000000000000, -1.000000000000000000, 0.000000000000000000 ) ) ;
#21653=CARTESIAN_POINT ( 'NONE',  ( -1.878215178124998275, 26.00312499938549493, 12.25316411605951927 ) ) ;
#21659=EDGE_LOOP ( 'NONE', ( #11137, #14944, #15770 ) ) ;
#21663=CARTESIAN_POINT ( 'NONE',  ( -3.756430356250000546, 26.30312499938548854, 11.16877607737301226 ) ) ;
#21666=VECTOR ( 'NONE', #21640, 1000.000000000000000 ) ;
#21668=EDGE_CURVE ( 'NONE', #5730, #5871, #15260, .T. ) ;
#21677=CARTESIAN_POINT ( 'NONE',  ( -3.110308778861380574, 31.50000000000000000, 3.869115154270378110 ) ) ;
#21685=CARTESIAN_POINT ( 'NONE',  ( -3.999999999999996447, 29.18124999877097281, 6.690598923241487306 ) ) ;
#21686=CARTESIAN_POINT ( 'NONE',  ( 3.296389899763111586, 38.99989214654019776, 13.40352862988387095 ) ) ;
#21689=CARTESIAN_POINT ( 'NONE',  ( -5.438844394475538024, 38.59945611884848660, 6.711898833373152407 ) ) ;
#21699=CARTESIAN_POINT ( 'NONE',  ( -3.508499826075089700, 38.91217497027906802, 13.34949135706027690 ) ) ;
#21721=CYLINDRICAL_SURFACE ( 'NONE', #388, 0.5000000000000000000 ) ;
#21723=ORIENTED_EDGE ( 'NONE', *, *, #2128, .F. ) ;
#21728=ORIENTED_EDGE ( 'NONE', *, *, #19709, .T. ) ;
#21737=CARTESIAN_POINT ( 'NONE',  ( 4.000000000000001776, 29.50000000000000711, 8.999999999999992895 ) ) ;
#21746=CARTESIAN_POINT ( 'NONE',  ( 3.469446951953614189E-15, 35.50000000000000711, 8.999999999999992895 ) ) ;
#21756=CARTESIAN_POINT ( 'NONE',  ( -1.878215178124996498, 25.85312499938548925, 5.746835883940462963 ) ) ;
#21769=CARTESIAN_POINT ( 'NONE',  ( 1.878215178125005158, 28.81562499938548783, 5.746835883940462963 ) ) ;
#21772=CARTESIAN_POINT ( 'NONE',  ( 2.000000000000000000, 26.27500000000000568, 12.46410161513774817 ) ) ;
#21774=DIRECTION ( 'NONE',  ( -0.000000000000000000, -1.000000000000000000, -0.000000000000000000 ) ) ;
#21794=DIRECTION ( 'NONE',  ( -0.000000000000000000, 1.000000000000000000, -0.000000000000000000 ) ) ;
#21804=CARTESIAN_POINT ( 'NONE',  ( -1.878215178124996498, 29.45312499938548711, 5.746835883940462963 ) ) ;
#21813=CARTESIAN_POINT ( 'NONE',  ( 1.999999999999998224, 29.36874999877097636, 12.46410161513774817 ) ) ;
#21815=CARTESIAN_POINT ( 'NONE',  ( 5.112995299272250684E-15, 26.40624999877096712, 4.999999999999992006 ) ) ;
#21826=CARTESIAN_POINT ( 'NONE',  ( -4.000000000000000888, 29.25624999877096855, 11.30940107675849404 ) ) ;
#21837=CARTESIAN_POINT ( 'NONE',  ( -3.028776527127584828, 38.71721868403346178, 13.92618862263473289 ) ) ;
#21838=CIRCLE ( 'NONE', #958, 0.5000000000000004441 ) ;
#21839=CARTESIAN_POINT ( 'NONE',  ( -1.878215178124999829, 27.69062499938549138, 12.25316411605951927 ) ) ;
#21847=ADVANCED_FACE ( 'NONE', ( #2259 ), #13903, .T. ) ;
#21862=ORIENTED_EDGE ( 'NONE', *, *, #19056, .F. ) ;
#21878=DIRECTION ( 'NONE',  ( 0.000000000000000000, 0.000000000000000000, -1.000000000000000000 ) ) ;
#21886=CARTESIAN_POINT ( 'NONE',  ( 6.009258394948636914E-15, 29.10624999877097352, 4.381197846482986158 ) ) ;
#21895=CARTESIAN_POINT ( 'NONE',  ( -4.000000000000000000, 26.06874999877097210, 8.999999999999992895 ) ) ;
#21897=CARTESIAN_POINT ( 'NONE',  ( 3.526711513754840599, 38.89679573513954125, 4.645898033750303746 ) ) ;
#21899=CARTESIAN_POINT ( 'NONE',  ( -1.878215178124998275, 27.24062499938548854, 12.25316411605951927 ) ) ;
#21901=CARTESIAN_POINT ( 'NONE',  ( 0.3338636427494953152, 38.86740601410824070, 3.377184973053767969 ) ) ;
#21903=CARTESIAN_POINT ( 'NONE',  ( 4.000000000000005329, 28.18750000000000711, 6.690598923241489970 ) ) ;
#21909=FACE_OUTER_BOUND ( 'NONE', #18410, .T. ) ;
#21918=CARTESIAN_POINT ( 'NONE',  ( 1.878215178125001605, 27.87812499938548783, 12.25316411605952283 ) ) ;
#21925=ORIENTED_EDGE ( 'NONE', *, *, #204, .T. ) ;
#21929=CARTESIAN_POINT ( 'NONE',  ( -1.878215178124996498, 25.74062499938548854, 5.746835883940462963 ) ) ;
#21933=DIRECTION ( 'NONE',  ( 0.000000000000000000, 0.000000000000000000, 1.000000000000000000 ) ) ;
#21944=CARTESIAN_POINT ( 'NONE',  ( 5.706339097771728319, 38.63519838069890966, 7.645898033751371337 ) ) ;
#21946=DIRECTION ( 'NONE',  ( 0.000000000000000000, 0.000000000000000000, 1.000000000000000000 ) ) ;
#21963=CARTESIAN_POINT ( 'NONE',  ( -3.756430356249996105, 26.67812499938548854, 6.831223922626973533 ) ) ;
#21964=EDGE_CURVE ( 'NONE', #5871, #17035, #5400, .T. ) ;
#21970=B_SPLINE_CURVE_WITH_KNOTS ( 'NONE', 3,
 ( #23663, #13487, #5741, #21837, #6009, #13990, #21454, #4040, #3533, #11505, #13720, #21699, #3786, #20368, #20646, #18430 ),
 .UNSPECIFIED., .F., .F.,
 ( 4, 2, 2, 2, 2, 2, 2, 4 ),
 ( 2.789812635117653453E-07, 0.0002322844908107169664, 0.0004642900003579222032, 0.0006962955099051274400, 0.0009283010194523326226, 0.001160306528999537805, 0.001392312038546742988, 0.001856323057641153353 ),
 .UNSPECIFIED. ) ;
#21985=( BOUNDED_CURVE ( )  B_SPLINE_CURVE ( 2, ( #23399, #19590, #3643, #4032, #9795, #5733, #13984, #1950, #1695 ),
 .UNSPECIFIED., .F., .F. ) 
 B_SPLINE_CURVE_WITH_KNOTS ( ( 3, 2, 2, 2, 3 ),
 ( 0.6750000000000000444, 0.6833333333333333481, 0.6999999999999999556, 0.7166666666666666741, 0.7249999999999999778 ),
 .UNSPECIFIED. ) 
 CURVE ( )  GEOMETRIC_REPRESENTATION_ITEM ( )  RATIONAL_B_SPLINE_CURVE ( ( 0.9330127018922194093, 0.9330127018922198534, 1.000000000000000000, 0.8660254037844387076, 1.000000000000000000, 0.8660254037844387076, 1.000000000000000000, 0.9330127018922194093, 0.9330127018922194093 ) ) 
 REPRESENTATION_ITEM ( '' )  );
#21987=CARTESIAN_POINT ( 'NONE',  ( 0.000000000000000000, 29.78124999877097423, 12.99999999999999289 ) ) ;
#22008=CARTESIAN_POINT ( 'NONE',  ( 1.878215178125001605, 26.52812499938548640, 12.25316411605952283 ) ) ;
#22009=EDGE_LOOP ( 'NONE', ( #14409, #19320, #1411, #5523 ) ) ;
#22018=ADVANCED_FACE ( 'NONE', ( #4857 ), #8924, .T. ) ;
#22038=CARTESIAN_POINT ( 'NONE',  ( -3.756430356250000546, 28.21562499938548996, 11.16877607737301048 ) ) ;
#22046=CARTESIAN_POINT ( 'NONE',  ( -2.003086131649545506E-15, 27.27812499938548640, 13.33755215474602984 ) ) ;
#22054=CARTESIAN_POINT ( 'NONE',  ( 6.938893903907228378E-15, 31.50000000000000000, 2.999999999999992450 ) ) ;
#22065=CARTESIAN_POINT ( 'NONE',  ( -1.071796769724485232, 26.03259618943233988, 4.999999999999992006 ) ) ;
#22075=ORIENTED_EDGE ( 'NONE', *, *, #15359, .T. ) ;
#22077=EDGE_LOOP ( 'NONE', ( #16791, #3779, #5933, #22311, #19498, #8255, #17019, #18898, #4723, #16865, #6782, #21862, #12696, #4934, #19768, #166, #7325, #23811, #1241, #3941, #8526, #9442, #12428, #2846 ) ) ;
#22079=CARTESIAN_POINT ( 'NONE',  ( -1.878215178124998275, 26.30312499938548854, 5.746835883940462963 ) ) ;
#22083=CARTESIAN_POINT ( 'NONE',  ( -1.878215178124996498, 27.09062499938548996, 5.746835883940462963 ) ) ;
#22117=AXIS2_PLACEMENT_3D ( 'NONE', #5981, #17630, #21933 ) ;
#22138=CARTESIAN_POINT ( 'NONE',  ( 3.756430356250002323, 25.66562499938548925, 11.16877607737301226 ) ) ;
#22150=CARTESIAN_POINT ( 'NONE',  ( -0.4995657836784084815, 38.49999999999999289, 14.97916666666665897 ) ) ;
#22156=FACE_OUTER_BOUND ( 'NONE', #20174, .T. ) ;
#22158=CARTESIAN_POINT ( 'NONE',  ( -3.999999999999999556, 28.41250000000000142, 11.30940107675849404 ) ) ;
#22159=CIRCLE ( 'NONE', #23823, 6.000000000000000000 ) ;
#22160=DIRECTION ( 'NONE',  ( 0.000000000000000000, 0.000000000000000000, -1.000000000000000000 ) ) ;
#22173=ORIENTED_EDGE ( 'NONE', *, *, #5089, .T. ) ;
#22176=CARTESIAN_POINT ( 'NONE',  ( 3.756430356250004987, 27.95312499938548711, 8.999999999999992895 ) ) ;
#22186=CARTESIAN_POINT ( 'NONE',  ( 8.012344526598182026E-15, 28.85312499938549280, 4.662447845253954171 ) ) ;
#22195=VECTOR ( 'NONE', #6494, 1000.000000000000000 ) ;
#22198=CARTESIAN_POINT ( 'NONE',  ( -1.071796769724485676, 26.61115380933863861, 12.99999999999999467 ) ) ;
#22216=EDGE_CURVE ( 'NONE', #16526, #15841, #2574, .T. ) ;
#22222=CARTESIAN_POINT ( 'NONE',  ( 3.756430356250004543, 25.74062499938548498, 6.831223922626973533 ) ) ;
#22225=CARTESIAN_POINT ( 'NONE',  ( -3.999999999999996447, 28.86250000000000071, 11.30940107675849404 ) ) ;
#22235=DIRECTION ( 'NONE',  ( 0.000000000000000000, 0.000000000000000000, 1.000000000000000000 ) ) ;
#22260=CARTESIAN_POINT ( 'NONE',  ( 4.000000000000007105, 25.93750000000000711, 6.690598923241489970 ) ) ;
#22274=CARTESIAN_POINT ( 'NONE',  ( -1.878215178124999829, 27.80312499938548854, 12.25316411605951927 ) ) ;
#22278=VERTEX_POINT ( 'NONE', #17880 ) ;
#22291=CARTESIAN_POINT ( 'NONE',  ( 4.000000000000000888, 28.63750000000000639, 6.690598923241489970 ) ) ;
#22294=EDGE_CURVE ( 'NONE', #15214, #10411, #15872, .T. ) ;
#22299=CARTESIAN_POINT ( 'NONE',  ( -0.2827178117968723869, 38.91165577845126222, 3.418461308658551356 ) ) ;
#22305=CARTESIAN_POINT ( 'NONE',  ( -3.756430356249994329, 26.86562499938548498, 11.16877607737301048 ) ) ;
#22311=ORIENTED_EDGE ( 'NONE', *, *, #20840, .F. ) ;
#22314=CARTESIAN_POINT ( 'NONE',  ( 3.756430356250006319, 26.97812499938548569, 6.831223922626973533 ) ) ;
#22317=CARTESIAN_POINT ( 'NONE',  ( 2.000000000000005329, 26.42500000000000426, 5.535898384862238508 ) ) ;
#22326=ORIENTED_EDGE ( 'NONE', *, *, #15640, .F. ) ;
#22327=CYLINDRICAL_SURFACE ( 'NONE', #948, 6.000000000000000888 ) ;
#22342=ORIENTED_EDGE ( 'NONE', *, *, #18426, .F. ) ;
#22345=CARTESIAN_POINT ( 'NONE',  ( 3.756430356250000546, 26.56562499938548783, 11.16877607737301226 ) ) ;
#22355=CARTESIAN_POINT ( 'NONE',  ( -3.526711513754876570, 31.50000000000000000, 4.145898033750337497 ) ) ;
#22358=CARTESIAN_POINT ( 'NONE',  ( 5.112995299272250684E-15, 27.36250000000000426, 4.999999999999992006 ) ) ;
#22360=ADVANCED_FACE ( 'NONE', ( #8464 ), #24283, .F. ) ;
#22369=EDGE_LOOP ( 'NONE', ( #7062, #20506, #7064, #2878 ) ) ;
#22370=VERTEX_POINT ( 'NONE', #24414 ) ;
#22373=VERTEX_POINT ( 'NONE', #16312 ) ;
#22395=VERTEX_POINT ( 'NONE', #2821 ) ;
#22396=CARTESIAN_POINT ( 'NONE',  ( 8.012344526598182026E-15, 28.06562499938548783, 4.662447845253954171 ) ) ;
#22404=CARTESIAN_POINT ( 'NONE',  ( -1.071796769724484344, 25.97634618820330843, 4.999999999999992006 ) ) ;
#22406=CARTESIAN_POINT ( 'NONE',  ( -0.1556054994193453167, 38.97851006807007224, 14.51964528620012551 ) ) ;
#22416=FACE_OUTER_BOUND ( 'NONE', #2664, .T. ) ;
#22426=CARTESIAN_POINT ( 'NONE',  ( -3.756430356249997882, 28.62812499938548783, 8.999999999999992895 ) ) ;
#22437=CARTESIAN_POINT ( 'NONE',  ( -1.878215178124998275, 26.79062499938548569, 12.25316411605951927 ) ) ;
#22458=CARTESIAN_POINT ( 'NONE',  ( 5.706339097771728319, 38.63519838069890966, 7.645898033751371337 ) ) ;
#22459=LINE ( 'NONE', #127, #22784 ) ;
#22461=EDGE_CURVE ( 'NONE', #4270, #5730, #10593, .T. ) ;
#22465=EDGE_CURVE ( 'NONE', #16533, #12207, #13268, .T. ) ;
#22472=CARTESIAN_POINT ( 'NONE',  ( 1.878215178125003382, 25.32812499938548356, 5.746835883940462963 ) ) ;
#22473=EDGE_CURVE ( 'NONE', #3500, #21315, #15038, .T. ) ;
#22474=VECTOR ( 'NONE', #23426, 1000.000000000000000 ) ;
#22492=ORIENTED_EDGE ( 'NONE', *, *, #23531, .F. ) ;
#22501=ORIENTED_EDGE ( 'NONE', *, *, #9867, .T. ) ;
#22508=EDGE_CURVE ( 'NONE', #12276, #17574, #10874, .T. ) ;
#22515=SHAPE_REPRESENTATION ( 'bezel locker', ( #21036 ), #21481 ) ;
#22523=CARTESIAN_POINT ( 'NONE',  ( 1.394453263437886604E-15, 28.88124999877097210, 12.99999999999999289 ) ) ;
#22529=CARTESIAN_POINT ( 'NONE',  ( -3.756430356249994773, 28.17812499938548854, 8.999999999999992895 ) ) ;
#22548=CARTESIAN_POINT ( 'NONE',  ( -1.999999999999994893, 28.75000000000000355, 5.535898384862237620 ) ) ;
#22554=AXIS2_PLACEMENT_3D ( 'NONE', #10787, #14476, #16452 ) ;
#22560=CARTESIAN_POINT ( 'NONE',  ( 5.732828587490932826, 38.61000136877622424, 10.35167381828165567 ) ) ;
#22572=ADVANCED_FACE ( 'NONE', ( #19647 ), #23699, .T. ) ;
#22574=VERTEX_POINT ( 'NONE', #19783 ) ;
#22576=CARTESIAN_POINT ( 'NONE',  ( -3.756430356249994773, 27.16562499938548214, 8.999999999999992895 ) ) ;
#22580=CARTESIAN_POINT ( 'NONE',  ( -1.878215178124998275, 27.24062499938548854, 12.25316411605951927 ) ) ;
#22582=CIRCLE ( 'NONE', #20061, 6.000000000000000000 ) ;
#22585=ADVANCED_FACE ( 'NONE', ( #10095 ), #4075, .T. ) ;
#22593=CARTESIAN_POINT ( 'NONE',  ( -0.4995657836784015426, 38.49999999999999289, 3.020833333333323267 ) ) ;
#22597=ORIENTED_EDGE ( 'NONE', *, *, #10109, .F. ) ;
#22607=AXIS2_PLACEMENT_3D ( 'NONE', #11445, #8980, #5048 ) ;
#22608=ORIENTED_EDGE ( 'NONE', *, *, #21964, .F. ) ;
#22613=CARTESIAN_POINT ( 'NONE',  ( 8.012344526598182026E-15, 25.81562499938549138, 4.662447845253954171 ) ) ;
#22637=VERTEX_POINT ( 'NONE', #15861 ) ;
#22672=CARTESIAN_POINT ( 'NONE',  ( 4.006172263299091013E-15, 28.96562499938548996, 4.662447845253954171 ) ) ;
#22699=ADVANCED_FACE ( 'NONE', ( #4465 ), #20408, .T. ) ;
#22704=CARTESIAN_POINT ( 'NONE',  ( -1.878215178124999829, 29.15312499938549351, 12.25316411605951927 ) ) ;
#22711=CARTESIAN_POINT ( 'NONE',  ( -3.756430356249996105, 29.37812499938548427, 6.831223922626973533 ) ) ;
#22712=CARTESIAN_POINT ( 'NONE',  ( 3.756430356250002323, 26.52812499938548640, 6.831223922626973533 ) ) ;
#22714=CARTESIAN_POINT ( 'NONE',  ( 5.112995299272250684E-15, 25.56250000000000711, 4.999999999999992006 ) ) ;
#22715=CARTESIAN_POINT ( 'NONE',  ( -1.878215178124994722, 26.64062499938549067, 5.746835883940462963 ) ) ;
#22730=EDGE_CURVE ( 'NONE', #8768, #19772, #4747, .T. ) ;
#22734=LINE ( 'NONE', #6771, #19680 ) ;
#22746=CARTESIAN_POINT ( 'NONE',  ( -1.878215178124996498, 27.65312499938548996, 5.746835883940462963 ) ) ;
#22784=VECTOR ( 'NONE', #12392, 1000.000000000000000 ) ;
#22795=CARTESIAN_POINT ( 'NONE',  ( 1.878215178125008489, 27.57812499938549422, 5.746835883940462963 ) ) ;
#22800=EDGE_CURVE ( 'NONE', #18677, #855, #13732, .T. ) ;
#22810=B_SPLINE_CURVE_WITH_KNOTS ( 'NONE', 3,
 ( #5817, #25702, #25826, #12088, #16035, #11956 ),
 .UNSPECIFIED., .F., .F.,
 ( 4, 2, 4 ),
 ( 2.789812639092967010E-07, 0.0002989033495849343454, 0.0005975277179059593300 ),
 .UNSPECIFIED. ) ;
#22837=CARTESIAN_POINT ( 'NONE',  ( 2.000000000000000000, 25.82500000000000639, 12.46410161513774817 ) ) ;
#22852=CARTESIAN_POINT ( 'NONE',  ( -1.999999999999994893, 25.54374999877097352, 5.535898384862237620 ) ) ;
#22865=CARTESIAN_POINT ( 'NONE',  ( 8.012344526598182026E-15, 28.51562499938549067, 4.662447845253954171 ) ) ;
#22888=ORIENTED_EDGE ( 'NONE', *, *, #3482, .F. ) ;
#22896=DIRECTION ( 'NONE',  ( 0.000000000000000000, 0.000000000000000000, -1.000000000000000000 ) ) ;
#22902=EDGE_CURVE ( 'NONE', #25109, #11111, #22159, .T. ) ;
#22927=CARTESIAN_POINT ( 'NONE',  ( 3.756430356250004987, 25.25312499938548427, 8.999999999999992895 ) ) ;
#22943=CARTESIAN_POINT ( 'NONE',  ( -3.999999999999994671, 26.93124999877097281, 6.690598923241487306 ) ) ;
#22948=AXIS2_PLACEMENT_3D ( 'NONE', #25557, #23847, #1496 ) ;
#22951=CARTESIAN_POINT ( 'NONE',  ( 6.009258394948636914E-15, 29.41562499938548925, 4.662447845253954171 ) ) ;
#22961=CARTESIAN_POINT ( 'NONE',  ( 3.469446951953614189E-15, 39.50000000000000000, 8.999999999999992895 ) ) ;
#22962=CARTESIAN_POINT ( 'NONE',  ( 2.003086131649545506E-15, 29.07812499938549067, 13.33755215474602984 ) ) ;
#22966=CARTESIAN_POINT ( 'NONE',  ( 4.000000000000002665, 29.03124999877096712, 6.690598923241489970 ) ) ;
#22970=EDGE_CURVE ( 'NONE', #2251, #7412, #6139, .T. ) ;
#22971=DIRECTION ( 'NONE',  ( 0.000000000000000000, 1.000000000000000000, 0.000000000000000000 ) ) ;
#22985=ORIENTED_EDGE ( 'NONE', *, *, #5952, .T. ) ;
#22998=CARTESIAN_POINT ( 'NONE',  ( 1.878215178125001605, 28.77812499938549351, 12.25316411605952283 ) ) ;
#23003=( NAMED_UNIT ( * ) SI_UNIT ( $, .STERADIAN. ) SOLID_ANGLE_UNIT ( ) );
#23010=PRODUCT_DEFINITION_CONTEXT ( 'detailed design', #13960, 'design' ) ;
#23019=CARTESIAN_POINT ( 'NONE',  ( 3.469446951953614189E-15, 35.50000000000000711, 8.999999999999992895 ) ) ;
#23022=DIRECTION ( 'NONE',  ( -0.000000000000000000, 1.000000000000000000, -0.000000000000000000 ) ) ;
#23024=CARTESIAN_POINT ( 'NONE',  ( -5.312859100616741159, 38.96936022227531282, 7.461857399205459096 ) ) ;
#23050=EDGE_CURVE ( 'NONE', #5730, #17641, #14123, .T. ) ;
#23057=DIRECTION ( 'NONE',  ( 0.000000000000000000, 0.000000000000000000, -1.000000000000000000 ) ) ;
#23082=CARTESIAN_POINT ( 'NONE',  ( -3.999999999999996447, 27.00624999877096855, 11.30940107675849404 ) ) ;
#23098=CARTESIAN_POINT ( 'NONE',  ( 3.756430356250002323, 25.62812499938548072, 6.831223922626973533 ) ) ;
#23102=CARTESIAN_POINT ( 'NONE',  ( -3.999999999999999556, 25.18750000000000711, 6.690598923241487306 ) ) ;
#23104=DIRECTION ( 'NONE',  ( -0.000000000000000000, -1.000000000000000000, -0.000000000000000000 ) ) ;
#23108=CARTESIAN_POINT ( 'NONE',  ( -1.999999999999998224, 27.04374999877097352, 12.46410161513774639 ) ) ;
#23116=ORIENTED_EDGE ( 'NONE', *, *, #3296, .T. ) ;
#23129=CARTESIAN_POINT ( 'NONE',  ( 3.756430356250004543, 28.89062499938549067, 6.831223922626973533 ) ) ;
#23137=CARTESIAN_POINT ( 'NONE',  ( 4.648177544792955347E-16, 28.93750000000000355, 12.99999999999999289 ) ) ;
#23140=CARTESIAN_POINT ( 'NONE',  ( 5.706339097770929847, 29.50000000000000000, 10.85410196624966517 ) ) ;
#23158=CARTESIAN_POINT ( 'NONE',  ( 5.840899737312978957, 34.50000000000000000, 10.37254881831474052 ) ) ;
#23174=CARTESIAN_POINT ( 'NONE',  ( -3.999999999999996447, 25.22500000000000497, 8.999999999999992895 ) ) ;
#23191=CARTESIAN_POINT ( 'NONE',  ( 3.469446951953614189E-15, 31.50000000000000000, 8.999999999999992895 ) ) ;
#23198=CARTESIAN_POINT ( 'NONE',  ( 4.000000000000002665, 27.23124999877097352, 6.690598923241489970 ) ) ;
#23212=CARTESIAN_POINT ( 'NONE',  ( -3.756430356249998326, 29.45312499938549422, 11.16877607737301226 ) ) ;
#23213=CARTESIAN_POINT ( 'NONE',  ( 1.878215178124998275, 25.51562499938548711, 12.25316411605952283 ) ) ;
#23216=CARTESIAN_POINT ( 'NONE',  ( -1.878215178124998275, 29.49062499938548854, 12.25316411605951927 ) ) ;
#23243=ORIENTED_EDGE ( 'NONE', *, *, #22473, .T. ) ;
#23245=CARTESIAN_POINT ( 'NONE',  ( 2.003086131649545506E-15, 27.39062499938549067, 13.33755215474602984 ) ) ;
#23248=FILL_AREA_STYLE ('',( #11348 ) ) ;
#23249=LINE ( 'NONE', #7686, #12203 ) ;
#23254=CARTESIAN_POINT ( 'NONE',  ( 3.469446951953614189E-15, 35.50000000000000711, 4.999999999999992006 ) ) ;
#23256=EDGE_CURVE ( 'NONE', #19772, #21027, #3790, .T. ) ;
#23265=CARTESIAN_POINT ( 'NONE',  ( -1.878215178124996498, 29.45312499938548711, 5.746835883940462963 ) ) ;
#23272=ORIENTED_EDGE ( 'NONE', *, *, #21964, .T. ) ;
#23291=EDGE_CURVE ( 'NONE', #4422, #7506, #8504, .T. ) ;
#23303=ORIENTED_EDGE ( 'NONE', *, *, #19537, .F. ) ;
#23305=EDGE_CURVE ( 'NONE', #19496, #15395, #6936, .T. ) ;
#23318=ORIENTED_EDGE ( 'NONE', *, *, #2378, .F. ) ;
#23320=CARTESIAN_POINT ( 'NONE',  ( 2.000000000000000000, 27.11874999877097281, 12.46410161513774817 ) ) ;
#23329=EDGE_LOOP ( 'NONE', ( #25551, #1350, #11617, #18292 ) ) ;
#23333=AXIS2_PLACEMENT_3D ( 'NONE', #6470, #8176, #2679 ) ;
#23337=CARTESIAN_POINT ( 'NONE',  ( 8.012344526598182026E-15, 28.85312499938549280, 4.662447845253954171 ) ) ;
#23339=CARTESIAN_POINT ( 'NONE',  ( -3.999999999999999556, 25.26250000000000284, 11.30940107675849404 ) ) ;
#23341=VECTOR ( 'NONE', #7493, 1000.000000000000114 ) ;
#23356=CARTESIAN_POINT ( 'NONE',  ( -5.706339097770898761, 31.50000000000000000, 10.85410196624973800 ) ) ;
#23361=B_SPLINE_CURVE_WITH_KNOTS ( 'NONE', 3,
 ( #18866, #8932, #13112, #19368 ),
 .UNSPECIFIED., .F., .F.,
 ( 4, 4 ),
 ( 2.789812634830972505E-07, 0.0001914289244202972522 ),
 .UNSPECIFIED. ) ;
#23374=CARTESIAN_POINT ( 'NONE',  ( -3.756430356249996105, 25.77812499938548640, 6.831223922626973533 ) ) ;
#23378=VECTOR ( 'NONE', #20669, 1000.000000000000000 ) ;
#23382=CARTESIAN_POINT ( 'NONE',  ( -9.296355089585910693E-16, 26.91250000000000497, 4.999999999999991118 ) ) ;
#23397=CARTESIAN_POINT ( 'NONE',  ( -1.878215178124999829, 29.15312499938549351, 12.25316411605951927 ) ) ;
#23398=CARTESIAN_POINT ( 'NONE',  ( -5.706339097770933400, 38.63519838069944967, 7.645898033750358813 ) ) ;
#23399=CARTESIAN_POINT ( 'NONE',  ( 1.487416814333745711E-14, 28.43124999877096926, 12.99999999999999289 ) ) ;
#23410=EDGE_CURVE ( 'NONE', #19215, #930, #19767, .T. ) ;
#23426=DIRECTION ( 'NONE',  ( 0.000000000000000000, 1.000000000000000000, -0.000000000000000000 ) ) ;
#23440=EDGE_CURVE ( 'NONE', #16647, #11238, #8079, .T. ) ;
#23447=CARTESIAN_POINT ( 'NONE',  ( 3.959305671612554781E-15, 25.00000000000000000, 12.99999999999999289 ) ) ;
#23458=CARTESIAN_POINT ( 'NONE',  ( 4.000000000000000888, 27.15624999877097423, 11.30940107675849760 ) ) ;
#23459=AXIS2_PLACEMENT_3D ( 'NONE', #25374, #23552, #11636 ) ;
#23471=CARTESIAN_POINT ( 'NONE',  ( 0.3342655765624356068, 38.86701176172695682, 14.62318542138302213 ) ) ;
#23474=CARTESIAN_POINT ( 'NONE',  ( -1.878215178124996498, 28.44062499938548783, 5.746835883940462963 ) ) ;
#23477=CARTESIAN_POINT ( 'NONE',  ( -3.999999999999996447, 26.16250000000000497, 11.30940107675849404 ) ) ;
#23497=LINE ( 'NONE', #23742, #1284 ) ;
#23507=CARTESIAN_POINT ( 'NONE',  ( 3.756430356250000546, 25.55312499938548498, 11.16877607737301226 ) ) ;
#23518=CARTESIAN_POINT ( 'NONE',  ( 3.918623196469464443, 38.49999999999999289, 4.456389954662531849 ) ) ;
#23529=VERTEX_POINT ( 'NONE', #8081 ) ;
#23531=EDGE_CURVE ( 'NONE', #22278, #18677, #14235, .T. ) ;
#23532=CARTESIAN_POINT ( 'NONE',  ( -5.201695249984999769, 38.97584342600590190, 7.139037124126438094 ) ) ;
#23540=CARTESIAN_POINT ( 'NONE',  ( 5.577813053751546416E-15, 25.33750000000000924, 12.99999999999999289 ) ) ;
#23544=CARTESIAN_POINT ( 'NONE',  ( -3.756430356249996549, 25.36562499938548854, 8.999999999999992895 ) ) ;
#23551=CARTESIAN_POINT ( 'NONE',  ( -3.110308778861273105, 34.50000000000000000, 14.13088484572967118 ) ) ;
#23552=DIRECTION ( 'NONE',  ( 0.000000000000000000, 1.000000000000000000, 0.000000000000000000 ) ) ;
#23567=EDGE_CURVE ( 'NONE', #10619, #7410, #12985, .T. ) ;
#23585=DIRECTION ( 'NONE',  ( 0.000000000000000000, -1.000000000000000000, 0.000000000000000000 ) ) ;
#23589=CARTESIAN_POINT ( 'NONE',  ( -4.000000000000001776, 29.21874999877097068, 8.999999999999992895 ) ) ;
#23590=( BOUNDED_CURVE ( )  B_SPLINE_CURVE ( 2, ( #21507, #5801, #11557, #1625, #9357 ),
 .UNSPECIFIED., .F., .F. ) 
 B_SPLINE_CURVE_WITH_KNOTS ( ( 3, 2, 3 ),
 ( 0.000000000000000000, 0.01666666666666666644, 0.02500000000000000486 ),
 .UNSPECIFIED. ) 
 CURVE ( )  GEOMETRIC_REPRESENTATION_ITEM ( )  RATIONAL_B_SPLINE_CURVE ( ( 1.000000000000000000, 0.8660254037844387076, 1.000000000000000000, 0.9330127018922194093, 0.9330127018922194093 ) ) 
 REPRESENTATION_ITEM ( '' )  );
#23603=CARTESIAN_POINT ( 'NONE',  ( -3.756430356249996549, 27.61562499938548143, 8.999999999999992895 ) ) ;
#23604=CARTESIAN_POINT ( 'NONE',  ( 0.4995657836784154204, 38.49999999999999289, 3.020833333333325044 ) ) ;
#23605=CARTESIAN_POINT ( 'NONE',  ( 4.000000000000005329, 27.73750000000000782, 6.690598923241489970 ) ) ;
#23608=CARTESIAN_POINT ( 'NONE',  ( -0.4995657836784057060, 31.50000000000000000, 3.020833333333325044 ) ) ;
#23610=CARTESIAN_POINT ( 'NONE',  ( -3.999999999999998224, 26.96874999877097068, 8.999999999999992895 ) ) ;
#23619=CARTESIAN_POINT ( 'NONE',  ( 1.071796769724492782, 25.75134618820331056, 12.99999999999999467 ) ) ;
#23623=CARTESIAN_POINT ( 'NONE',  ( -1.878215178124998275, 25.55312499938549564, 12.25316411605951927 ) ) ;
#23633=CARTESIAN_POINT ( 'NONE',  ( -1.878215178124996498, 26.19062499938548783, 5.746835883940462963 ) ) ;
#23636=CARTESIAN_POINT ( 'NONE',  ( -1.999999999999998224, 28.39374999877097139, 12.46410161513774639 ) ) ;
#23640=CARTESIAN_POINT ( 'NONE',  ( 5.532151103383248447, 31.50000000000000000, 11.32277940608563149 ) ) ;
#23651=CARTESIAN_POINT ( 'NONE',  ( 3.110308778861349932, 38.49999999999999289, 14.13088484572963033 ) ) ;
#23663=CARTESIAN_POINT ( 'NONE',  ( -3.110308778861273105, 38.49999999999999289, 14.13088484572967118 ) ) ;
#23675=CARTESIAN_POINT ( 'NONE',  ( 4.000000000000002665, 27.66249999999999787, 11.30940107675849760 ) ) ;
#23678=CARTESIAN_POINT ( 'NONE',  ( -5.840899737312955864, 38.49999999999999289, 10.37254881831481512 ) ) ;
#23699=CYLINDRICAL_SURFACE ( 'NONE', #18821, 4.000000000000000000 ) ;
#23703=CARTESIAN_POINT ( 'NONE',  ( 1.071796769724496334, 28.24240381056767291, 4.999999999999992895 ) ) ;
#23706=CARTESIAN_POINT ( 'NONE',  ( 4.000000000000005329, 29.48124999877097707, 6.690598923241489970 ) ) ;
#23709=CARTESIAN_POINT ( 'NONE',  ( -1.071796769724487897, 29.36740381056767291, 12.99999999999999289 ) ) ;
#23715=ORIENTED_EDGE ( 'NONE', *, *, #9365, .F. ) ;
#23718=CARTESIAN_POINT ( 'NONE',  ( -1.878215178124999829, 29.04062499938549280, 12.25316411605951927 ) ) ;
#23721=CARTESIAN_POINT ( 'NONE',  ( 0.000000000000000000, 26.68750000000000711, 13.61880215351699874 ) ) ;
#23737=FACE_OUTER_BOUND ( 'NONE', #1054, .T. ) ;
#23742=CARTESIAN_POINT ( 'NONE',  ( -3.526711513754876570, 29.50000000000000000, 4.645898033750338385 ) ) ;
#23751=CARTESIAN_POINT ( 'NONE',  ( -3.756430356249996105, 29.49062499938548854, 6.831223922626973533 ) ) ;
#23758=VECTOR ( 'NONE', #7701, 1000.000000000000000 ) ;
#23772=EDGE_CURVE ( 'NONE', #4730, #13467, #10932, .T. ) ;
#23783=ORIENTED_EDGE ( 'NONE', *, *, #204, .F. ) ;
#23790=CARTESIAN_POINT ( 'NONE',  ( 3.756430356250002323, 27.35312499938548569, 11.16877607737301226 ) ) ;
#23804=CARTESIAN_POINT ( 'NONE',  ( 3.469446951953614189E-15, 31.50000000000000000, 8.999999999999992895 ) ) ;
#23811=ORIENTED_EDGE ( 'NONE', *, *, #11708, .F. ) ;
#23817=DIRECTION ( 'NONE',  ( 0.000000000000000000, 1.000000000000000000, 0.000000000000000000 ) ) ;
#23823=AXIS2_PLACEMENT_3D ( 'NONE', #5246, #15197, #19481 ) ;
#23841=VERTEX_POINT ( 'NONE', #10664 ) ;
#23844=CARTESIAN_POINT ( 'NONE',  ( 1.878215178125008489, 26.22812499938548925, 5.746835883940462963 ) ) ;
#23847=DIRECTION ( 'NONE',  ( 0.000000000000000000, 1.000000000000000000, 0.000000000000000000 ) ) ;
#23858=CARTESIAN_POINT ( 'NONE',  ( 3.068624420619302740, 38.57523615308659970, 3.931826694835521163 ) ) ;
#23860=CARTESIAN_POINT ( 'NONE',  ( 3.756430356250004099, 28.70312499938548356, 11.16877607737301403 ) ) ;
#23864=CARTESIAN_POINT ( 'NONE',  ( 2.000000000000000000, 28.07500000000000995, 12.46410161513774817 ) ) ;
#23884=VERTEX_POINT ( 'NONE', #1514 ) ;
#23893=CARTESIAN_POINT ( 'NONE',  ( 3.469446951953614189E-15, 38.49999999999999289, 8.999999999999992895 ) ) ;
#23895=CARTESIAN_POINT ( 'NONE',  ( 1.878215178125003382, 26.11562499938548854, 5.746835883940462963 ) ) ;
#23903=CARTESIAN_POINT ( 'NONE',  ( 4.000000000000002665, 29.40624999877096357, 11.30940107675849760 ) ) ;
#23909=CARTESIAN_POINT ( 'NONE',  ( -5.480138960579897578, 38.55544002051693298, 11.30344864665788585 ) ) ;
#23912=CARTESIAN_POINT ( 'NONE',  ( 0.000000000000000000, 29.50000000000000000, 14.99999999999999289 ) ) ;
#23914=CARTESIAN_POINT ( 'NONE',  ( 3.469446951953614189E-15, 35.50000000000000711, 4.999999999999992006 ) ) ;
#23928=( NAMED_UNIT ( * ) PLANE_ANGLE_UNIT ( ) SI_UNIT ( $, .RADIAN. ) );
#23929=CARTESIAN_POINT ( 'NONE',  ( 6.009258394948636914E-15, 26.15312499938548640, 4.662447845253954171 ) ) ;
#23946=DIRECTION ( 'NONE',  ( 0.000000000000000000, 0.000000000000000000, 1.000000000000000000 ) ) ;
#23950=ORIENTED_EDGE ( 'NONE', *, *, #6026, .T. ) ;
#23957=ORIENTED_EDGE ( 'NONE', *, *, #14943, .T. ) ;
#23959=EDGE_CURVE ( 'NONE', #20975, #7296, #17603, .T. ) ;
#23965=CARTESIAN_POINT ( 'NONE',  ( 4.648177544792955347E-16, 25.78750000000000497, 12.99999999999999289 ) ) ;
#23968=CARTESIAN_POINT ( 'NONE',  ( -1.999999999999996669, 27.49374999877097636, 12.46410161513774639 ) ) ;
#23974=DIRECTION ( 'NONE',  ( 0.000000000000000000, 0.000000000000000000, 1.000000000000000000 ) ) ;
#23978=CARTESIAN_POINT ( 'NONE',  ( -3.756430356249996105, 26.41562499938548925, 11.16877607737301226 ) ) ;
#23982=CARTESIAN_POINT ( 'NONE',  ( 4.648177544792954952E-15, 28.26250000000000284, 4.999999999999992006 ) ) ;
#23983=ORIENTED_EDGE ( 'NONE', *, *, #4769, .F. ) ;
#23988=CARTESIAN_POINT ( 'NONE',  ( -1.878215178124994722, 29.34062499938548640, 5.746835883940462963 ) ) ;
#23992=CARTESIAN_POINT ( 'NONE',  ( 4.000000000000007105, 29.08750000000000568, 6.690598923241489970 ) ) ;
#24001=DIRECTION ( 'NONE',  ( 0.000000000000000000, 0.000000000000000000, 1.000000000000000000 ) ) ;
#24008=CARTESIAN_POINT ( 'NONE',  ( 6.009258394948636914E-15, 27.61562499938548854, 4.662447845253954171 ) ) ;
#24015=DIRECTION ( 'NONE',  ( -0.000000000000000000, -1.000000000000000000, -0.000000000000000000 ) ) ;
#24016=CARTESIAN_POINT ( 'NONE',  ( -1.878215178124996498, 27.09062499938548996, 5.746835883940462963 ) ) ;
#24039=CARTESIAN_POINT ( 'NONE',  ( 1.071796769724493226, 26.65134618820330914, 12.99999999999999112 ) ) ;
#24048=CARTESIAN_POINT ( 'NONE',  ( 3.756430356250003211, 26.15312499938548996, 8.999999999999992895 ) ) ;
#24049=CARTESIAN_POINT ( 'NONE',  ( 3.756430356250004543, 27.87812499938548783, 6.831223922626973533 ) ) ;
#24069=CARTESIAN_POINT ( 'NONE',  ( -1.071796769724489451, 26.93259618943234202, 4.999999999999992895 ) ) ;
#24071=ORIENTED_EDGE ( 'NONE', *, *, #14564, .T. ) ;
#24085=DIRECTION ( 'NONE',  ( 0.000000000000000000, -1.000000000000000000, 0.000000000000000000 ) ) ;
#24096=CARTESIAN_POINT ( 'NONE',  ( -3.756430356249996549, 25.47812499938548925, 8.999999999999992895 ) ) ;
#24102=CARTESIAN_POINT ( 'NONE',  ( -1.071796769724489895, 28.46740381056767433, 12.99999999999999289 ) ) ;
#24106=CARTESIAN_POINT ( 'NONE',  ( -0.2821657309629640453, 38.91194779626417954, 14.58126831647290444 ) ) ;
#24107=( BOUNDED_CURVE ( )  B_SPLINE_CURVE ( 2, ( #200, #8171, #24111, #4629, #14709, #16806, #6584, #12610, #24504 ),
 .UNSPECIFIED., .F., .F. ) 
 B_SPLINE_CURVE_WITH_KNOTS ( ( 3, 2, 2, 2, 3 ),
 ( 0.3250000000000000111, 0.3333333333333333148, 0.3499999999999999778, 0.3666666666666666408, 0.3750000000000000000 ),
 .UNSPECIFIED. ) 
 CURVE ( )  GEOMETRIC_REPRESENTATION_ITEM ( )  RATIONAL_B_SPLINE_CURVE ( ( 0.9330127018922194093, 0.9330127018922196314, 1.000000000000000000, 0.8660254037844387076, 1.000000000000000000, 0.8660254037844387076, 1.000000000000000000, 0.9330127018922194093, 0.9330127018922194093 ) ) 
 REPRESENTATION_ITEM ( '' )  );
#24109=CYLINDRICAL_SURFACE ( 'NONE', #5567, 6.000000000000000888 ) ;
#24111=CARTESIAN_POINT ( 'NONE',  ( -1.999999999999996669, 26.50000000000000355, 5.535898384862237620 ) ) ;
#24112=CARTESIAN_POINT ( 'NONE',  ( -1.999999999999994893, 29.20000000000000284, 5.535898384862237620 ) ) ;
#24113=( BOUNDED_CURVE ( )  B_SPLINE_CURVE ( 2, ( #17030, #10735, #17164, #813, #18607, #11010, #18721, #5135, #12585 ),
 .UNSPECIFIED., .F., .F. ) 
 B_SPLINE_CURVE_WITH_KNOTS ( ( 3, 2, 2, 2, 3 ),
 ( 0.9250000000000000444, 0.9333333333333333481, 0.9499999999999999556, 0.9666666666666666741, 0.9749999999999999778 ),
 .UNSPECIFIED. ) 
 CURVE ( )  GEOMETRIC_REPRESENTATION_ITEM ( )  RATIONAL_B_SPLINE_CURVE ( ( 0.9330127018922194093, 0.9330127018922198534, 1.000000000000000000, 0.8660254037844387076, 1.000000000000000000, 0.8660254037844387076, 1.000000000000000000, 0.9330127018922194093, 0.9330127018922194093 ) ) 
 REPRESENTATION_ITEM ( '' )  );
#24123=CARTESIAN_POINT ( 'NONE',  ( 5.787458694563957451, 38.55544002051694008, 10.35761576072610168 ) ) ;
#24127=CARTESIAN_POINT ( 'NONE',  ( 1.878215178125001605, 27.42812499938548854, 12.25316411605952283 ) ) ;
#24130=CARTESIAN_POINT ( 'NONE',  ( 7.437084071668728555E-15, 27.13750000000000639, 12.99999999999999112 ) ) ;
#24136=CARTESIAN_POINT ( 'NONE',  ( 4.006172263299091013E-15, 28.40312499938548996, 4.662447845253954171 ) ) ;
#24141=DIRECTION ( 'NONE',  ( 0.000000000000000000, 0.000000000000000000, 1.000000000000000000 ) ) ;
#24146=LINE ( 'NONE', #24635, #21255 ) ;
#24163=DIRECTION ( 'NONE',  ( 0.000000000000000000, 0.000000000000000000, 1.000000000000000000 ) ) ;
#24169=VECTOR ( 'NONE', #19425, 1000.000000000000000 ) ;
#24177=CARTESIAN_POINT ( 'NONE',  ( 3.756430356250004987, 26.49062499938548854, 8.999999999999992895 ) ) ;
#24178=CARTESIAN_POINT ( 'NONE',  ( -3.999999999999996447, 28.78750000000000497, 6.690598923241487306 ) ) ;
#24201=ORIENTED_EDGE ( 'NONE', *, *, #22730, .F. ) ;
#24203=ORIENTED_EDGE ( 'NONE', *, *, #4774, .F. ) ;
#24226=CARTESIAN_POINT ( 'NONE',  ( 4.000000000000005329, 25.43124999877097636, 6.690598923241489970 ) ) ;
#24230=CARTESIAN_POINT ( 'NONE',  ( 3.756430356250003211, 27.05312499938548854, 8.999999999999992895 ) ) ;
#24231=AXIS2_PLACEMENT_3D ( 'NONE', #10479, #18478, #21878 ) ;
#24233=LINE ( 'NONE', #2525, #12087 ) ;
#24248=CARTESIAN_POINT ( 'NONE',  ( 4.000000000000007105, 28.60000000000000497, 8.999999999999992895 ) ) ;
#24254=PRODUCT ( 'bezel locker', 'bezel locker', '', ( #3091 ) ) ;
#24255=CARTESIAN_POINT ( 'NONE',  ( 6.009258394948636914E-15, 25.95624999877097139, 4.381197846482986158 ) ) ;
#24263=CARTESIAN_POINT ( 'NONE',  ( 0.000000000000000000, 28.29062499938549280, 13.33755215474603162 ) ) ;
#24274=CARTESIAN_POINT ( 'NONE',  ( 1.878215178125001605, 29.11562499938549209, 12.25316411605952283 ) ) ;
#24276=CARTESIAN_POINT ( 'NONE',  ( -3.110308778861381462, 38.49999999999999289, 3.869115154270378554 ) ) ;
#24283=CYLINDRICAL_SURFACE ( 'NONE', #22554, 0.5000000000000004441 ) ;
#24284=CARTESIAN_POINT ( 'NONE',  ( 3.469446951953614189E-15, 39.50000000000000000, 8.999999999999992895 ) ) ;
#24293=CARTESIAN_POINT ( 'NONE',  ( 5.208121455455055226, 38.94679493378507118, 7.072325123572092309 ) ) ;
#24297=CIRCLE ( 'NONE', #20106, 6.000000000000000000 ) ;
#24310=EDGE_LOOP ( 'NONE', ( #24403, #14249, #960, #13244 ) ) ;
#24312=CARTESIAN_POINT ( 'NONE',  ( -1.878215178124999829, 26.45312499938549422, 12.25316411605951927 ) ) ;
#24318=DIRECTION ( 'NONE',  ( 0.000000000000000000, 1.000000000000000000, 0.000000000000000000 ) ) ;
#24328=EDGE_CURVE ( 'NONE', #855, #12364, #20538, .T. ) ;
#24329=DIRECTION ( 'NONE',  ( -0.000000000000000000, 1.000000000000000000, -0.000000000000000000 ) ) ;
#24344=ORIENTED_EDGE ( 'NONE', *, *, #6636, .T. ) ;
#24356=( BOUNDED_SURFACE ( )  B_SPLINE_SURFACE ( 1, 2, ( 
 ( #9301, #17287, #25367, #7330, #21325, #9422, #23544, #7717, #15437, #25120, #17403, #3535, #11506, #19477, #21573, #3652, #25636, #14597, #15820, #2699, #139, #8705, #14738, #12149, #735, #6749, #6133, #23929, #2226, #16692, #8112, #19860, #17909, #17787, #10659, #10056, #24177, #24662, #15960, #3921, #22715, #21963, #4660, #7975, #18651, #20124, #25876, #6011, #4795, #10183, #1843, #1959, #22083, #19744, #19984, #4041, #22580, #9806, #9922, #23790, #13992, #12642, #12008, #25753, #7836, #5880, #2088, #13864, #21839, #20614, #264, #18055, #16087, #24049, #14118, #4170, #6609, #18182, #8230, #11891, #16206, #5049, #20867, #867, #1116, #7001, #1389, #3088, #7389, #6879, #15369, #7274, #10924, #14985, #7140, #19035, #25190, #9091, #13279, #14863, #19290, #24923, #11054, #24798, #1000, #22962, #9231, #15250, #17078, #25052, #2960, #17219, #21127, #3334, #9363, #13032, #23216, #15127, #21251, #5300, #11311 ),
 ( #12889, #17347, #25311, #20742, #11172, #23102, #5185, #23339, #18916, #12771, #8981, #8847, #2819, #16957, #13160, #21011, #10782, #3204, #19155, #18778, #1248, #16835, #22837, #4911, #19803, #16028, #11565, #1511, #13797, #19533, #11698, #23477, #21393, #9989, #21772, #2022, #17458, #1633, #3714, #19416, #25429, #11446, #25570, #9611, #17983, #23721, #3857, #25819, #7516, #7901, #5430, #15510, #7778, #19675, #9480, #13419, #5564, #13548, #17725, #73, #15757, #3473, #1903, #21511, #25696, #5810, #11833, #8047, #3592, #17593, #1778, #7652, #15639, #23605, #9866, #11950, #9745, #5683, #13662, #21635, #17849, #15892, #23864, #5949, #13935, #21903, #3984, #19920, #8294, #4103, #2405, #22158, #16151, #20188, #2159, #4241, #24248, #22291, #8172, #14451, #22548, #10364, #12081, #322, #14568, #6464, #8433, #12220, #16279, #23992, #2539, #6074, #24112, #20056, #8680, #20312, #4630, #18363, #14186, #20441, #14057 ) ),
 .UNSPECIFIED., .F., .F., .F. ) 
 B_SPLINE_SURFACE_WITH_KNOTS ( ( 2, 2 ),
 ( 3, 2, 2, 2, 2, 2, 2, 2, 2, 2, 2, 2, 2, 2, 2, 2, 2, 2, 2, 2, 2, 2, 2, 2, 2, 2, 2, 2, 2, 2, 2, 2, 2, 2, 2, 2, 2, 2, 2, 2, 2, 2, 2, 2, 2, 2, 2, 2, 2, 2, 2, 2, 2, 2, 2, 2, 2, 2, 2, 2, 3 ),
 ( 0.000000000000000000, 1.000000000000000000 ),
 ( 0.000000000000000000, 0.01666666666666666644, 0.03333333333333333287, 0.05000000000000000278, 0.06666666666666666574, 0.08333333333333332871, 0.1000000000000000056, 0.1166666666666666685, 0.1333333333333333315, 0.1499999999999999944, 0.1666666666666666574, 0.1833333333333333204, 0.2000000000000000111, 0.2166666666666666741, 0.2333333333333333370, 0.2500000000000000000, 0.2666666666666666630, 0.2833333333333333259, 0.2999999999999999889, 0.3166666666666666519, 0.3333333333333333148, 0.3499999999999999778, 0.3666666666666666408, 0.3833333333333333592, 0.4000000000000000222, 0.4166666666666666852, 0.4333333333333333481, 0.4500000000000000111, 0.4666666666666666741, 0.4833333333333333370, 0.5000000000000000000, 0.5166666666666667185, 0.5333333333333333259, 0.5500000000000000444, 0.5666666666666666519, 0.5833333333333333703, 0.5999999999999999778, 0.6166666666666666963, 0.6333333333333333037, 0.6500000000000000222, 0.6666666666666666297, 0.6833333333333333481, 0.6999999999999999556, 0.7166666666666666741, 0.7333333333333332815, 0.7500000000000000000, 0.7666666666666667185, 0.7833333333333333259, 0.8000000000000000444, 0.8166666666666666519, 0.8333333333333333703, 0.8499999999999999778, 0.8666666666666666963, 0.8833333333333333037, 0.9000000000000000222, 0.9166666666666666297, 0.9333333333333333481, 0.9499999999999999556, 0.9666666666666666741, 0.9833333333333332815, 1.000000000000000000 ),
 .UNSPECIFIED. ) 
 GEOMETRIC_REPRESENTATION_ITEM ( )  RATIONAL_B_SPLINE_SURFACE ( (
 ( 1.000000000000000000, 0.8660254037844387076, 1.000000000000000000, 0.8660254037844387076, 1.000000000000000000, 0.8660254037844387076, 1.000000000000000000, 0.8660254037844387076, 1.000000000000000000, 0.8660254037844387076, 1.000000000000000000, 0.8660254037844387076, 1.000000000000000000, 0.8660254037844387076, 1.000000000000000000, 0.8660254037844387076, 1.000000000000000000, 0.8660254037844387076, 1.000000000000000000, 0.8660254037844387076, 1.000000000000000000, 0.8660254037844387076, 1.000000000000000000, 0.8660254037844387076, 1.000000000000000000, 0.8660254037844387076, 1.000000000000000000, 0.8660254037844387076, 1.000000000000000000, 0.8660254037844387076, 1.000000000000000000, 0.8660254037844387076, 1.000000000000000000, 0.8660254037844387076, 1.000000000000000000, 0.8660254037844387076, 1.000000000000000000, 0.8660254037844387076, 1.000000000000000000, 0.8660254037844387076, 1.000000000000000000, 0.8660254037844387076, 1.000000000000000000, 0.8660254037844387076, 1.000000000000000000, 0.8660254037844387076, 1.000000000000000000, 0.8660254037844387076, 1.000000000000000000, 0.8660254037844387076, 1.000000000000000000, 0.8660254037844387076, 1.000000000000000000, 0.8660254037844387076, 1.000000000000000000, 0.8660254037844387076, 1.000000000000000000, 0.8660254037844387076, 1.000000000000000000, 0.8660254037844387076, 1.000000000000000000, 0.8660254037844387076, 1.000000000000000000, 0.8660254037844387076, 1.000000000000000000, 0.8660254037844387076, 1.000000000000000000, 0.8660254037844387076, 1.000000000000000000, 0.8660254037844387076, 1.000000000000000000, 0.8660254037844387076, 1.000000000000000000, 0.8660254037844387076, 1.000000000000000000, 0.8660254037844387076, 1.000000000000000000, 0.8660254037844387076, 1.000000000000000000, 0.8660254037844387076, 1.000000000000000000, 0.8660254037844387076, 1.000000000000000000, 0.8660254037844387076, 1.000000000000000000, 0.8660254037844387076, 1.000000000000000000, 0.8660254037844387076, 1.000000000000000000, 0.8660254037844387076, 1.000000000000000000, 0.8660254037844387076, 1.000000000000000000, 0.8660254037844387076, 1.000000000000000000, 0.8660254037844387076, 1.000000000000000000, 0.8660254037844387076, 1.000000000000000000, 0.8660254037844387076, 1.000000000000000000, 0.8660254037844387076, 1.000000000000000000, 0.8660254037844387076, 1.000000000000000000, 0.8660254037844387076, 1.000000000000000000, 0.8660254037844387076, 1.000000000000000000, 0.8660254037844387076, 1.000000000000000000, 0.8660254037844387076, 1.000000000000000000, 0.8660254037844387076, 1.000000000000000000, 0.8660254037844387076, 1.000000000000000000, 0.8660254037844387076, 1.000000000000000000, 0.8660254037844387076, 1.000000000000000000),
 ( 1.000000000000000000, 0.8660254037844387076, 1.000000000000000000, 0.8660254037844387076, 1.000000000000000000, 0.8660254037844387076, 1.000000000000000000, 0.8660254037844387076, 1.000000000000000000, 0.8660254037844387076, 1.000000000000000000, 0.8660254037844387076, 1.000000000000000000, 0.8660254037844387076, 1.000000000000000000, 0.8660254037844387076, 1.000000000000000000, 0.8660254037844387076, 1.000000000000000000, 0.8660254037844387076, 1.000000000000000000, 0.8660254037844387076, 1.000000000000000000, 0.8660254037844387076, 1.000000000000000000, 0.8660254037844387076, 1.000000000000000000, 0.8660254037844387076, 1.000000000000000000, 0.8660254037844387076, 1.000000000000000000, 0.8660254037844387076, 1.000000000000000000, 0.8660254037844387076, 1.000000000000000000, 0.8660254037844387076, 1.000000000000000000, 0.8660254037844387076, 1.000000000000000000, 0.8660254037844387076, 1.000000000000000000, 0.8660254037844387076, 1.000000000000000000, 0.8660254037844387076, 1.000000000000000000, 0.8660254037844387076, 1.000000000000000000, 0.8660254037844387076, 1.000000000000000000, 0.8660254037844387076, 1.000000000000000000, 0.8660254037844387076, 1.000000000000000000, 0.8660254037844387076, 1.000000000000000000, 0.8660254037844387076, 1.000000000000000000, 0.8660254037844387076, 1.000000000000000000, 0.8660254037844387076, 1.000000000000000000, 0.8660254037844387076, 1.000000000000000000, 0.8660254037844387076, 1.000000000000000000, 0.8660254037844387076, 1.000000000000000000, 0.8660254037844387076, 1.000000000000000000, 0.8660254037844387076, 1.000000000000000000, 0.8660254037844387076, 1.000000000000000000, 0.8660254037844387076, 1.000000000000000000, 0.8660254037844387076, 1.000000000000000000, 0.8660254037844387076, 1.000000000000000000, 0.8660254037844387076, 1.000000000000000000, 0.8660254037844387076, 1.000000000000000000, 0.8660254037844387076, 1.000000000000000000, 0.8660254037844387076, 1.000000000000000000, 0.8660254037844387076, 1.000000000000000000, 0.8660254037844387076, 1.000000000000000000, 0.8660254037844387076, 1.000000000000000000, 0.8660254037844387076, 1.000000000000000000, 0.8660254037844387076, 1.000000000000000000, 0.8660254037844387076, 1.000000000000000000, 0.8660254037844387076, 1.000000000000000000, 0.8660254037844387076, 1.000000000000000000, 0.8660254037844387076, 1.000000000000000000, 0.8660254037844387076, 1.000000000000000000, 0.8660254037844387076, 1.000000000000000000, 0.8660254037844387076, 1.000000000000000000, 0.8660254037844387076, 1.000000000000000000, 0.8660254037844387076, 1.000000000000000000, 0.8660254037844387076, 1.000000000000000000, 0.8660254037844387076, 1.000000000000000000, 0.8660254037844387076, 1.000000000000000000) ) ) 
 REPRESENTATION_ITEM ( '' )  SURFACE ( )  );
#24370=ORIENTED_EDGE ( 'NONE', *, *, #23291, .T. ) ;
#24371=CARTESIAN_POINT ( 'NONE',  ( 0.000000000000000000, 28.29062499938548925, 13.33755215474602984 ) ) ;
#24384=DIRECTION ( 'NONE',  ( -0.000000000000000000, -1.000000000000000000, -0.000000000000000000 ) ) ;
#24401=CARTESIAN_POINT ( 'NONE',  ( -1.878215178124996498, 28.55312499938548854, 5.746835883940462963 ) ) ;
#24403=ORIENTED_EDGE ( 'NONE', *, *, #16826, .T. ) ;
#24404=DIRECTION ( 'NONE',  ( -0.000000000000000000, -1.000000000000000000, -0.000000000000000000 ) ) ;
#24411=CARTESIAN_POINT ( 'NONE',  ( -1.878215178124996498, 28.89062499938548711, 5.746835883940462963 ) ) ;
#24414=CARTESIAN_POINT ( 'NONE',  ( -5.706339097770933400, 38.63519838069944967, 7.645898033750358813 ) ) ;
#24435=( BOUNDED_CURVE ( )  B_SPLINE_CURVE ( 2, ( #23982, #20045, #2527, #20575, #4359, #18496, #12455, #24102, #10115 ),
 .UNSPECIFIED., .F., .F. ) 
 B_SPLINE_CURVE_WITH_KNOTS ( ( 3, 2, 2, 2, 3 ),
 ( 0.7249999999999999778, 0.7333333333333332815, 0.7500000000000000000, 0.7666666666666667185, 0.7750000000000000222 ),
 .UNSPECIFIED. ) 
 CURVE ( )  GEOMETRIC_REPRESENTATION_ITEM ( )  RATIONAL_B_SPLINE_CURVE ( ( 0.9330127018922194093, 0.9330127018922194093, 1.000000000000000000, 0.8660254037844387076, 1.000000000000000000, 0.8660254037844387076, 1.000000000000000000, 0.9330127018922194093, 0.9330127018922194093 ) ) 
 REPRESENTATION_ITEM ( '' )  );
#24452=DIRECTION ( 'NONE',  ( 0.000000000000000000, 0.000000000000000000, 1.000000000000000000 ) ) ;
#24461=AXIS2_PLACEMENT_3D ( 'NONE', #2885, #18592, #12711 ) ;
#24462=CARTESIAN_POINT ( 'NONE',  ( 4.000000000000002665, 27.68124999877097281, 6.690598923241489970 ) ) ;
#24466=ORIENTED_EDGE ( 'NONE', *, *, #23531, .T. ) ;
#24472=ORIENTED_EDGE ( 'NONE', *, *, #15099, .T. ) ;
#24488=CARTESIAN_POINT ( 'NONE',  ( -3.756430356249997882, 28.62812499938548783, 8.999999999999992895 ) ) ;
#24504=CARTESIAN_POINT ( 'NONE',  ( 4.648177544792955347E-16, 26.68750000000000711, 12.99999999999999289 ) ) ;
#24508=CYLINDRICAL_SURFACE ( 'NONE', #23333, 0.5000000000000004441 ) ;
#24509=CARTESIAN_POINT ( 'NONE',  ( -1.999999999999993117, 25.99374999877097281, 5.535898384862237620 ) ) ;
#24512=CARTESIAN_POINT ( 'NONE',  ( 4.000000000000003553, 25.39374999877097494, 8.999999999999992895 ) ) ;
#24516=CARTESIAN_POINT ( 'NONE',  ( -1.878215178124996498, 27.65312499938548996, 5.746835883940462963 ) ) ;
#24524=CARTESIAN_POINT ( 'NONE',  ( 0.000000000000000000, 28.62812499938549138, 13.33755215474602984 ) ) ;
#24531=CIRCLE ( 'NONE', #14117, 0.5000000000000004441 ) ;
#24556=CARTESIAN_POINT ( 'NONE',  ( 1.878215178124999829, 25.62812499938549138, 12.25316411605952283 ) ) ;
#24586=ORIENTED_EDGE ( 'NONE', *, *, #10394, .T. ) ;
#24600=EDGE_CURVE ( 'NONE', #12001, #1533, #13728, .T. ) ;
#24609=CARTESIAN_POINT ( 'NONE',  ( 1.071796769724494558, 25.48615380933863150, 4.999999999999992006 ) ) ;
#24613=CARTESIAN_POINT ( 'NONE',  ( 3.756430356250003211, 28.85312499938548569, 8.999999999999992895 ) ) ;
#24615=EDGE_LOOP ( 'NONE', ( #18049, #3529, #981, #797, #7680, #18319, #2425, #8187, #18320, #11154, #14073, #10140, #21723, #10461, #22492, #8770 ) ) ;
#24616=ORIENTED_EDGE ( 'NONE', *, *, #25507, .T. ) ;
#24617=DIRECTION ( 'NONE',  ( -0.000000000000000000, 1.000000000000000000, -0.000000000000000000 ) ) ;
#24635=CARTESIAN_POINT ( 'NONE',  ( 3.959305671612554781E-15, 35.50000000000000711, 12.99999999999999289 ) ) ;
#24638=CARTESIAN_POINT ( 'NONE',  ( -4.000000000000000000, 26.06874999877097210, 8.999999999999992895 ) ) ;
#24639=CARTESIAN_POINT ( 'NONE',  ( 3.756430356250004987, 29.75312499938549138, 8.999999999999992895 ) ) ;
#24653=VECTOR ( 'NONE', #5997, 1000.000000000000000 ) ;
#24659=CARTESIAN_POINT ( 'NONE',  ( 3.756430356250003211, 25.59062499938548285, 8.999999999999992895 ) ) ;
#24662=CARTESIAN_POINT ( 'NONE',  ( 3.756430356250002323, 26.52812499938548640, 6.831223922626973533 ) ) ;
#24668=CIRCLE ( 'NONE', #3369, 6.000000000000000000 ) ;
#24680=EDGE_CURVE ( 'NONE', #17275, #16526, #21435, .T. ) ;
#24693=ORIENTED_EDGE ( 'NONE', *, *, #604, .T. ) ;
#24698=CIRCLE ( 'NONE', #4640, 0.5000000000000004441 ) ;
#24699=CARTESIAN_POINT ( 'NONE',  ( 1.878215178125005158, 27.12812499938548783, 5.746835883940462963 ) ) ;
#24706=DIRECTION ( 'NONE',  ( 8.881784197001254296E-16, 0.000000000000000000, 1.000000000000000000 ) ) ;
#24721=ORIENTED_EDGE ( 'NONE', *, *, #14533, .T. ) ;
#24741=CARTESIAN_POINT ( 'NONE',  ( 3.959305671612554781E-15, 35.50000000000000711, 12.99999999999999289 ) ) ;
#24742=DIRECTION ( 'NONE',  ( 0.000000000000000000, 0.000000000000000000, 1.000000000000000000 ) ) ;
#24751=ADVANCED_FACE ( 'NONE', ( #7950 ), #22327, .T. ) ;
#24755=EDGE_LOOP ( 'NONE', ( #15538, #8138, #18083, #16978 ) ) ;
#24757=CARTESIAN_POINT ( 'NONE',  ( 3.756430356250004543, 27.01562499938549067, 11.16877607737301226 ) ) ;
#24770=VECTOR ( 'NONE', #20306, 1000.000000000000000 ) ;
#24776=CARTESIAN_POINT ( 'NONE',  ( 3.469446951953614189E-15, 35.50000000000000711, 8.999999999999992895 ) ) ;
#24778=ORIENTED_EDGE ( 'NONE', *, *, #19593, .F. ) ;
#24780=CARTESIAN_POINT ( 'NONE',  ( 2.000000000000003553, 25.91874999877097352, 5.535898384862238508 ) ) ;
#24795=CARTESIAN_POINT ( 'NONE',  ( -3.756430356250000546, 26.75312499938548783, 11.16877607737301048 ) ) ;
#24798=CARTESIAN_POINT ( 'NONE',  ( -3.756430356249996105, 29.00312499938548427, 11.16877607737301226 ) ) ;
#24818=DIRECTION ( 'NONE',  ( -0.000000000000000000, -1.000000000000000000, -0.000000000000000000 ) ) ;
#24833=CARTESIAN_POINT ( 'NONE',  ( -3.756430356249998326, 28.14062499938548356, 6.831223922626973533 ) ) ;
#24837=CARTESIAN_POINT ( 'NONE',  ( -3.020831617684079706, 38.79222141784235589, 4.157034316757149739 ) ) ;
#24856=VERTEX_POINT ( 'NONE', #25862 ) ;
#24858=ORIENTED_EDGE ( 'NONE', *, *, #23567, .F. ) ;
#24862=ORIENTED_EDGE ( 'NONE', *, *, #7234, .F. ) ;
#24866=EDGE_CURVE ( 'NONE', #11133, #15750, #13420, .T. ) ;
#24871=CYLINDRICAL_SURFACE ( 'NONE', #19706, 0.5000000000000004441 ) ;
#24894=DIRECTION ( 'NONE',  ( 0.000000000000000000, 0.000000000000000000, -1.000000000000000000 ) ) ;
#24908=CARTESIAN_POINT ( 'NONE',  ( 2.000000000000000000, 27.56874999877097210, 12.46410161513774817 ) ) ;
#24913=CARTESIAN_POINT ( 'NONE',  ( -1.878215178124998275, 29.60312499938548925, 12.25316411605951927 ) ) ;
#24921=CARTESIAN_POINT ( 'NONE',  ( -1.878215178124994722, 25.29062499938548925, 5.746835883940462963 ) ) ;
#24923=CARTESIAN_POINT ( 'NONE',  ( -3.756430356249996105, 28.92812499938548498, 6.831223922626973533 ) ) ;
#24925=CARTESIAN_POINT ( 'NONE',  ( 4.000000000000000888, 28.95624999877097494, 11.30940107675849760 ) ) ;
#24950=CARTESIAN_POINT ( 'NONE',  ( 1.878215178125008489, 27.57812499938549422, 5.746835883940462963 ) ) ;
#24956=( BOUNDED_CURVE ( )  B_SPLINE_CURVE ( 2, ( #1916, #23619, #1652, #13437, #7532, #19548, #9628, #9877, #15653 ),
 .UNSPECIFIED., .F., .F. ) 
 B_SPLINE_CURVE_WITH_KNOTS ( ( 3, 2, 2, 2, 3 ),
 ( 0.07500000000000001110, 0.08333333333333332871, 0.1000000000000000056, 0.1166666666666666685, 0.1250000000000000000 ),
 .UNSPECIFIED. ) 
 CURVE ( )  GEOMETRIC_REPRESENTATION_ITEM ( )  RATIONAL_B_SPLINE_CURVE ( ( 0.9330127018922192983, 0.9330127018922194093, 1.000000000000000000, 0.8660254037844387076, 1.000000000000000000, 0.8660254037844387076, 1.000000000000000000, 0.9330127018922194093, 0.9330127018922194093 ) ) 
 REPRESENTATION_ITEM ( '' )  );
#24968=DIRECTION ( 'NONE',  ( 0.000000000000000000, 0.000000000000000000, -1.000000000000000000 ) ) ;
#24989=CARTESIAN_POINT ( 'NONE',  ( -5.706339097770898761, 29.50000000000000000, 10.85410196624973800 ) ) ;
#24993=PRODUCT_DEFINITION ( 'UNKNOWN', '', #6035, #23010 ) ;
#25011=CARTESIAN_POINT ( 'NONE',  ( -3.999999999999999112, 27.90624999877098134, 11.30940107675849404 ) ) ;
#25023=DIRECTION ( 'NONE',  ( 0.000000000000000000, 0.000000000000000000, -1.000000000000000000 ) ) ;
#25029=ORIENTED_EDGE ( 'NONE', *, *, #7524, .T. ) ;
#25030=CARTESIAN_POINT ( 'NONE',  ( 2.000000000000005329, 28.61874999877097281, 5.535898384862238508 ) ) ;
#25039=CARTESIAN_POINT ( 'NONE',  ( -3.756430356249996549, 29.49062499938548854, 6.831223922626973533 ) ) ;
#25047=CARTESIAN_POINT ( 'NONE',  ( 3.756430356250004543, 29.22812499938548925, 6.831223922626973533 ) ) ;
#25048=CARTESIAN_POINT ( 'NONE',  ( -3.756430356249996549, 25.77812499938548285, 6.831223922626973533 ) ) ;
#25052=CARTESIAN_POINT ( 'NONE',  ( 3.756430356250004543, 29.22812499938548925, 6.831223922626973533 ) ) ;
#25060=LINE ( 'NONE', #9099, #24169 ) ;
#25085=CARTESIAN_POINT ( 'NONE',  ( -1.878215178124996498, 27.20312499938549067, 5.746835883940462963 ) ) ;
#25095=UNCERTAINTY_MEASURE_WITH_UNIT (LENGTH_MEASURE( 1.000000000000000082E-05 ), #6131, 'distance_accuracy_value', 'NONE');
#25108=CARTESIAN_POINT ( 'NONE',  ( -3.526711513754876570, 31.50000000000000000, 4.645898033750338385 ) ) ;
#25109=VERTEX_POINT ( 'NONE', #24276 ) ;
#25120=CARTESIAN_POINT ( 'NONE',  ( 4.006172263299091013E-15, 25.47812499938548925, 13.33755215474602984 ) ) ;
#25139=VERTEX_POINT ( 'NONE', #21123 ) ;
#25153=APPLICATION_CONTEXT ( 'automotive_design' ) ;
#25156=EDGE_CURVE ( 'NONE', #20504, #8259, #15784, .T. ) ;
#25164=DIRECTION ( 'NONE',  ( 0.000000000000000000, 1.000000000000000000, 0.000000000000000000 ) ) ;
#25170=EDGE_CURVE ( 'NONE', #20504, #6543, #12464, .T. ) ;
#25172=EDGE_LOOP ( 'NONE', ( #9155, #4790, #12125, #21728 ) ) ;
#25173=CARTESIAN_POINT ( 'NONE',  ( -1.999999999999994893, 26.89374999877097849, 5.535898384862237620 ) ) ;
#25187=CARTESIAN_POINT ( 'NONE',  ( 3.756430356250002323, 26.45312499938549067, 11.16877607737301403 ) ) ;
#25190=CARTESIAN_POINT ( 'NONE',  ( 3.756430356250003211, 28.74062499938548498, 8.999999999999992895 ) ) ;
#25194=DIRECTION ( 'NONE',  ( 0.000000000000000000, -1.000000000000000000, 0.000000000000000000 ) ) ;
#25218=ORIENTED_EDGE ( 'NONE', *, *, #8266, .T. ) ;
#25219=ORIENTED_EDGE ( 'NONE', *, *, #4335, .T. ) ;
#25221=CARTESIAN_POINT ( 'NONE',  ( -1.878215178124996498, 28.55312499938548854, 5.746835883940462963 ) ) ;
#25241=CARTESIAN_POINT ( 'NONE',  ( 1.878215178125003382, 29.67812499938549209, 12.25316411605952283 ) ) ;
#25244=EDGE_LOOP ( 'NONE', ( #9219, #2249, #3743, #10463 ) ) ;
#25252=CARTESIAN_POINT ( 'NONE',  ( -3.999999999999996447, 27.96250000000000568, 11.30940107675849404 ) ) ;
#25258=CARTESIAN_POINT ( 'NONE',  ( -9.296355089585909904E-15, 29.10624999877097352, 4.999999999999992006 ) ) ;
#25263=CARTESIAN_POINT ( 'NONE',  ( 3.526711513754818395, 31.50000000000000000, 4.145898033750289535 ) ) ;
#25270=ORIENTED_EDGE ( 'NONE', *, *, #10309, .T. ) ;
#25281=CARTESIAN_POINT ( 'NONE',  ( -3.918623196469422698, 31.50000000000000000, 13.54361004533748236 ) ) ;
#25286=ADVANCED_FACE ( 'NONE', ( #196 ), #24109, .T. ) ;
#25294=CARTESIAN_POINT ( 'NONE',  ( -4.000000000000000000, 27.86874999877096926, 8.999999999999992895 ) ) ;
#25309=CARTESIAN_POINT ( 'NONE',  ( -1.878215178124998275, 28.59062499938548640, 12.25316411605951927 ) ) ;
#25311=CARTESIAN_POINT ( 'NONE',  ( 2.000000000000005329, 25.07500000000000284, 5.535898384862238508 ) ) ;
#25325=ORIENTED_EDGE ( 'NONE', *, *, #17524, .F. ) ;
#25339=CARTESIAN_POINT ( 'NONE',  ( 1.878215178125006934, 25.21562499938548996, 5.746835883940462963 ) ) ;
#25342=CARTESIAN_POINT ( 'NONE',  ( 1.071796769724490783, 26.70759618943234059, 12.99999999999999467 ) ) ;
#25355=ORIENTED_EDGE ( 'NONE', *, *, #12800, .T. ) ;
#25362=ORIENTED_EDGE ( 'NONE', *, *, #5958, .F. ) ;
#25367=CARTESIAN_POINT ( 'NONE',  ( 1.878215178125006934, 25.21562499938548996, 5.746835883940462963 ) ) ;
#25374=CARTESIAN_POINT ( 'NONE',  ( 3.469446951953614189E-15, 31.50000000000000000, 8.999999999999992895 ) ) ;
#25410=CARTESIAN_POINT ( 'NONE',  ( 4.000000000000005329, 28.99374999877097281, 8.999999999999992895 ) ) ;
#25424=CARTESIAN_POINT ( 'NONE',  ( 0.4150711328764374874, 38.77044187147116361, 14.71462540935539920 ) ) ;
#25426=CARTESIAN_POINT ( 'NONE',  ( 3.756430356250003211, 26.94062499938548783, 8.999999999999992895 ) ) ;
#25429=CARTESIAN_POINT ( 'NONE',  ( -1.999999999999996669, 26.50000000000000355, 5.535898384862237620 ) ) ;
#25459=ORIENTED_EDGE ( 'NONE', *, *, #2241, .T. ) ;
#25461=CARTESIAN_POINT ( 'NONE',  ( 1.878215178125001605, 25.96562499938548996, 12.25316411605952283 ) ) ;
#25468=PRESENTATION_STYLE_ASSIGNMENT (( #21290 ) ) ;
#25485=DIRECTION ( 'NONE',  ( -0.000000000000000000, 1.000000000000000000, -0.000000000000000000 ) ) ;
#25486=CARTESIAN_POINT ( 'NONE',  ( 3.118766433812622196, 38.97868814324865383, 13.55653794922876898 ) ) ;
#25488=CARTESIAN_POINT ( 'NONE',  ( 1.878215178125001605, 29.22812499938549280, 12.25316411605952283 ) ) ;
#25495=VERTEX_POINT ( 'NONE', #3683 ) ;
#25501=CARTESIAN_POINT ( 'NONE',  ( 1.487416814333745711E-14, 28.03750000000001208, 12.99999999999999289 ) ) ;
#25507=EDGE_CURVE ( 'NONE', #3609, #1503, #11510, .T. ) ;
#25520=CARTESIAN_POINT ( 'NONE',  ( 1.487416814333745711E-14, 28.43124999877096926, 12.99999999999999289 ) ) ;
#25527=ORIENTED_EDGE ( 'NONE', *, *, #7524, .F. ) ;
#25534=VECTOR ( 'NONE', #11053, 1000.000000000000000 ) ;
#25551=ORIENTED_EDGE ( 'NONE', *, *, #25793, .F. ) ;
#25552=CARTESIAN_POINT ( 'NONE',  ( -1.999999999999996669, 29.29374999877097707, 12.46410161513774639 ) ) ;
#25556=ORIENTED_EDGE ( 'NONE', *, *, #25688, .F. ) ;
#25557=CARTESIAN_POINT ( 'NONE',  ( 3.469446951953614189E-15, 31.50000000000000000, 8.999999999999992895 ) ) ;
#25560=VERTEX_POINT ( 'NONE', #25281 ) ;
#25565=CARTESIAN_POINT ( 'NONE',  ( 3.041615118360314618, 38.64891868624847149, 4.001525436476169872 ) ) ;
#25567=CARTESIAN_POINT ( 'NONE',  ( -2.003086131649545506E-15, 27.27812499938548996, 13.33755215474603162 ) ) ;
#25570=CARTESIAN_POINT ( 'NONE',  ( -3.999999999999996447, 26.57500000000000639, 8.999999999999992895 ) ) ;
#25572=CARTESIAN_POINT ( 'NONE',  ( 3.469446951953614189E-15, 35.50000000000000711, 8.999999999999992895 ) ) ;
#25581=CARTESIAN_POINT ( 'NONE',  ( 1.071796769724489895, 27.10134618820330843, 12.99999999999999467 ) ) ;
#25588=CARTESIAN_POINT ( 'NONE',  ( -3.756430356249996549, 25.96562499938548996, 11.16877607737301048 ) ) ;
#25598=CARTESIAN_POINT ( 'NONE',  ( 6.009258394948636914E-15, 26.15312499938548640, 4.662447845253954171 ) ) ;
#25606=CARTESIAN_POINT ( 'NONE',  ( 2.000000000000000000, 26.72500000000000497, 12.46410161513774817 ) ) ;
#25636=CARTESIAN_POINT ( 'NONE',  ( -1.878215178124996498, 25.74062499938548854, 5.746835883940462963 ) ) ;
#25640=AXIS2_PLACEMENT_3D ( 'NONE', #22961, #16956, #11310 ) ;
#25654=CARTESIAN_POINT ( 'NONE',  ( -3.999999999999996447, 27.06250000000000000, 11.30940107675849404 ) ) ;
#25665=ORIENTED_EDGE ( 'NONE', *, *, #2801, .T. ) ;
#25673=CARTESIAN_POINT ( 'NONE',  ( 4.000000000000005329, 28.99374999877097281, 8.999999999999992895 ) ) ;
#25680=CARTESIAN_POINT ( 'NONE',  ( -1.999999999999994893, 29.59374999877097068, 5.535898384862237620 ) ) ;
#25688=EDGE_CURVE ( 'NONE', #20633, #4730, #13354, .T. ) ;
#25693=CARTESIAN_POINT ( 'NONE',  ( -1.878215178124996498, 27.09062499938548996, 5.746835883940462963 ) ) ;
#25694=B_SPLINE_CURVE_WITH_KNOTS ( 'NONE', 3,
 ( #23398, #3524, #7057, #15044, #23024, #5109, #17512, #23532, #17896, #5732, #16078, #11614, #21689, #13712 ),
 .UNSPECIFIED., .F., .F.,
 ( 4, 2, 2, 2, 2, 2, 4 ),
 ( 0.0001914289244202972522, 0.0006076524577255098137, 0.0008157642243781109987, 0.001023875991030711967, 0.001231987757683313152, 0.001440099524335914337, 0.001856323057641129934 ),
 .UNSPECIFIED. ) ;
#25696=CARTESIAN_POINT ( 'NONE',  ( -1.999999999999994893, 27.40000000000000213, 5.535898384862237620 ) ) ;
#25702=CARTESIAN_POINT ( 'NONE',  ( -3.874271733779039106, 38.57135925840245960, 4.512371625048121615 ) ) ;
#25716=ADVANCED_FACE ( 'NONE', ( #1320 ), #24356, .T. ) ;
#25722=CARTESIAN_POINT ( 'NONE',  ( -1.878215178124999829, 26.34062499938548996, 12.25316411605951927 ) ) ;
#25725=CARTESIAN_POINT ( 'NONE',  ( -1.071796769724483234, 28.41115380933863577, 12.99999999999999645 ) ) ;
#25734=CARTESIAN_POINT ( 'NONE',  ( -5.244799308578346420, 38.86679461760645182, 11.05583806265907754 ) ) ;
#25735=CARTESIAN_POINT ( 'NONE',  ( 5.312745220820863423, 38.96942687711479891, 7.461705451413530810 ) ) ;
#25738=CARTESIAN_POINT ( 'NONE',  ( -1.999999999999996669, 29.29374999877097707, 12.46410161513774639 ) ) ;
#25753=CARTESIAN_POINT ( 'NONE',  ( 6.009258394948636914E-15, 27.50312499938549138, 4.662447845253954171 ) ) ;
#25764=CARTESIAN_POINT ( 'NONE',  ( 2.000000000000003553, 26.36874999877097281, 5.535898384862238508 ) ) ;
#25791=AXIS2_PLACEMENT_3D ( 'NONE', #24776, #14226, #5984 ) ;
#25793=EDGE_CURVE ( 'NONE', #16647, #15841, #804, .T. ) ;
#25802=CARTESIAN_POINT ( 'NONE',  ( 1.878215178124999829, 25.62812499938549138, 12.25316411605952283 ) ) ;
#25815=CARTESIAN_POINT ( 'NONE',  ( -3.756430356249996549, 27.57812499938548356, 6.831223922626973533 ) ) ;
#25819=CARTESIAN_POINT ( 'NONE',  ( 4.000000000000002665, 26.76249999999999929, 11.30940107675849760 ) ) ;
#25825=AXIS2_PLACEMENT_3D ( 'NONE', #23912, #5994, #21946 ) ;
#25826=CARTESIAN_POINT ( 'NONE',  ( -3.819794567562884158, 38.64130726140524530, 4.557674856424296372 ) ) ;
#25832=DIRECTION ( 'NONE',  ( 0.000000000000000000, -1.000000000000000000, 0.000000000000000000 ) ) ;
#25833=CARTESIAN_POINT ( 'NONE',  ( -5.532151103383257329, 38.49999999999999289, 6.677220593914388935 ) ) ;
#25839=CARTESIAN_POINT ( 'NONE',  ( 1.878215178125001605, 26.07812499938549067, 12.25316411605952283 ) ) ;
#25847=CARTESIAN_POINT ( 'NONE',  ( 3.756430356250002323, 26.52812499938548640, 6.831223922626973533 ) ) ;
#25854=DIRECTION ( 'NONE',  ( -0.000000000000000000, -1.000000000000000000, -0.000000000000000000 ) ) ;
#25862=CARTESIAN_POINT ( 'NONE',  ( -3.526711513758413297, 38.89679573513893729, 4.645898033752330569 ) ) ;
#25869=CARTESIAN_POINT ( 'NONE',  ( -1.071796769724491671, 29.12634618820329990, 4.999999999999995559 ) ) ;
#25870=LINE ( 'NONE', #23914, #24653 ) ;
#25871=ORIENTED_EDGE ( 'NONE', *, *, #14564, .F. ) ;
#25872=CARTESIAN_POINT ( 'NONE',  ( 4.000000000000007105, 26.78124999877097068, 6.690598923241489970 ) ) ;
#25876=CARTESIAN_POINT ( 'NONE',  ( 1.878215178124998275, 26.86562499938548854, 12.25316411605952283 ) ) ;
#25901=COLOUR_RGB('Sky Blue',0.24,0.69,0.87);
#25902=FILL_AREA_STYLE_COLOUR('',#25901);
#25903=FILL_AREA_STYLE('',(#25902));
#25904=SURFACE_STYLE_FILL_AREA(#25903);
#25905=SURFACE_SIDE_STYLE('',(#25904));
#25906=SURFACE_STYLE_USAGE(.BOTH.,#25905);
#25907=PRESENTATION_STYLE_ASSIGNMENT((#25906));
ENDSEC;
END-ISO-10303-21;
